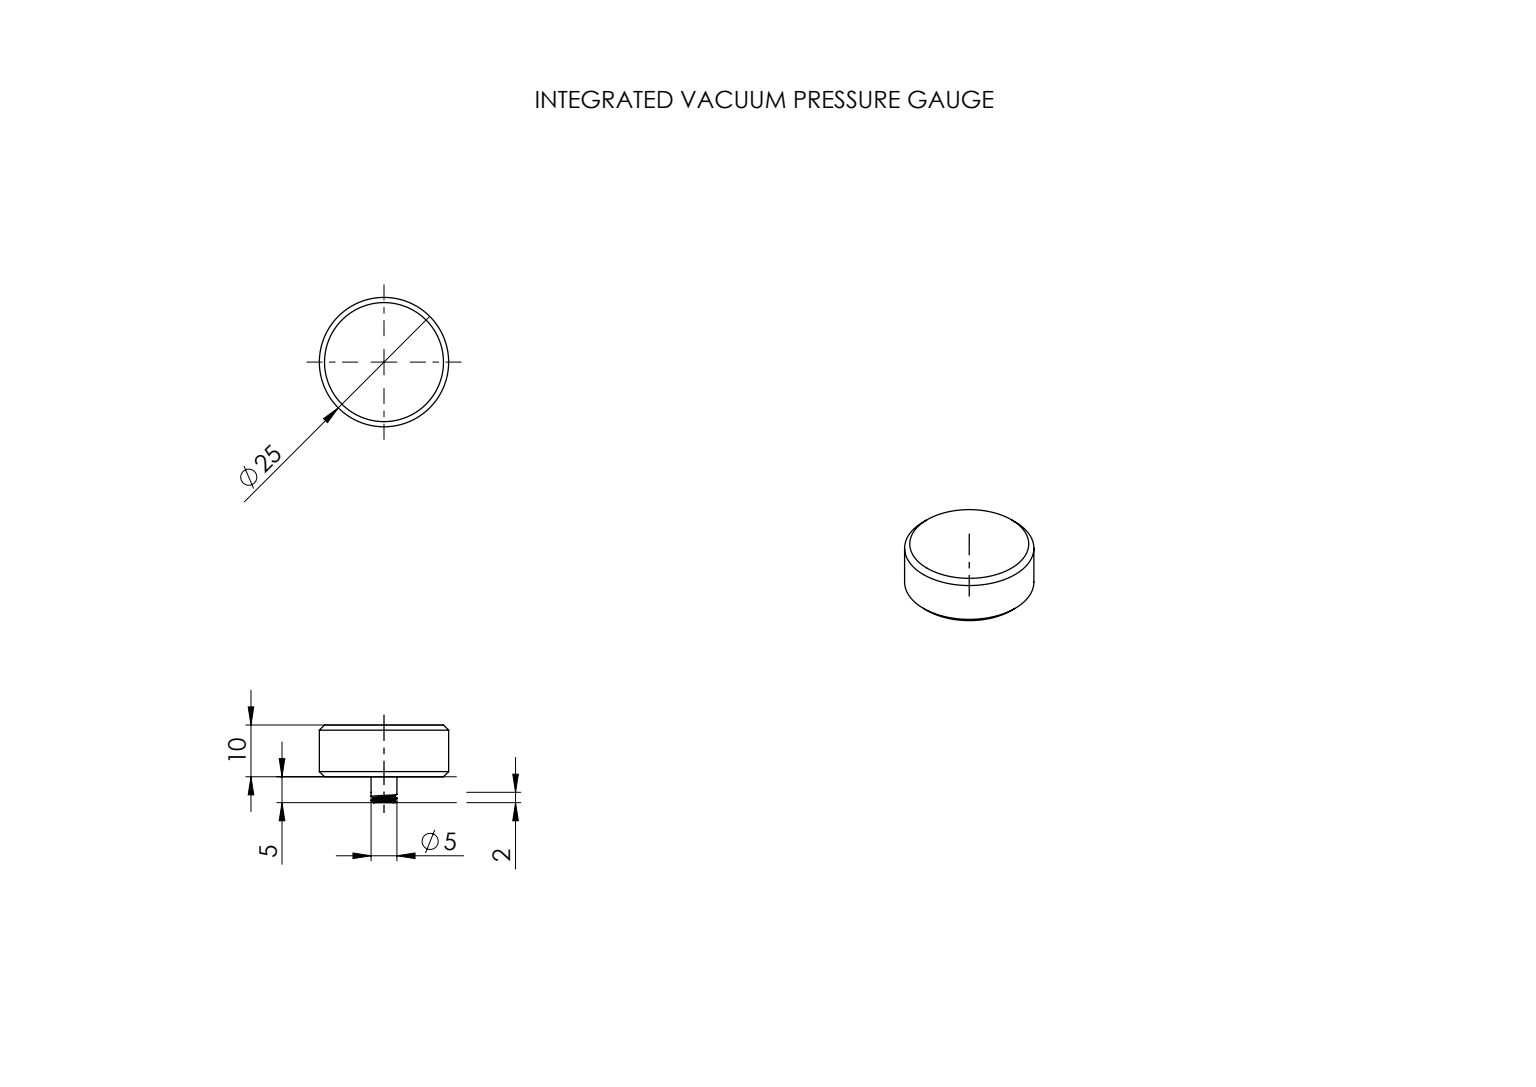
ISO-10303-21;
HEADER;
FILE_DESCRIPTION (('STEP AP214'),
    '1' );
FILE_NAME ('Integrated Vacuum Pressure Gauge.step',
    '2026-10-01T14:18:43',
    ( '' ),
    ( '' ),
    'SwSTEP 2.0',
    'SolidWorks 2026',
    '' );
FILE_SCHEMA (( 'AUTOMOTIVE_DESIGN' ));
ENDSEC;

DATA;
#26=CARTESIAN_POINT ( 'NONE',  ( 99.99999999999998579, 130.0000000000000000, 0.5000000000000034417 ) ) ;
#35=CARTESIAN_POINT ( 'NONE',  ( 102.0669872999999797, 124.3500000010924822, -9.794112055954760458E-15 ) ) ;
#135=CARTESIAN_POINT ( 'NONE',  ( 97.93294022916485631, 122.9999999999999858, -0.1348184704668160261 ) ) ;
#178=CARTESIAN_POINT ( 'NONE',  ( 101.4615807364564546, 124.2500000010924737, 1.461580736456455476 ) ) ;
#224=CYLINDRICAL_SURFACE ( 'NONE', #5646, 2.500000000000008882 ) ;
#256=ADVANCED_FACE ( 'NONE', ( #12743 ), #3942, .F. ) ;
#307=AXIS2_PLACEMENT_3D ( 'NONE', #10055, #1393, #9916 ) ;
#308=CARTESIAN_POINT ( 'NONE',  ( 97.93301270000000613, 124.7500000010924737, -9.540979117872439019E-15 ) ) ;
#319=CARTESIAN_POINT ( 'NONE',  ( 98.53841926354351699, 124.6500000010924651, -1.461580736456474794 ) ) ;
#324=EDGE_CURVE ( 'NONE', #25689, #13199, #21050, .T. ) ;
#329=ORIENTED_EDGE ( 'NONE', *, *, #20493, .F. ) ;
#336=AXIS2_PLACEMENT_3D ( 'NONE', #4217, #10471, #27744 ) ;
#342=EDGE_LOOP ( 'NONE', ( #1311, #13880, #16852, #27004 ) ) ;
#449=CARTESIAN_POINT ( 'NONE',  ( 97.93301269999999192, 124.7000000010924623, -0.8561741729129505041 ) ) ;
#463=CARTESIAN_POINT ( 'NONE',  ( 101.4615807364564546, 124.4500000010924765, -1.461580736456474794 ) ) ;
#487=VERTEX_POINT ( 'NONE', #17746 ) ;
#496=CARTESIAN_POINT ( 'NONE',  ( 97.50000000000000000, 124.9500000000000028, -1.035533905932742416 ) ) ;
#513=PLANE ( 'NONE',  #11990 ) ;
#550=CARTESIAN_POINT ( 'NONE',  ( 97.93301270000000613, 124.5500000010924850, -9.540979117872439019E-15 ) ) ;
#565=ORIENTED_EDGE ( 'NONE', *, *, #12281, .F. ) ;
#566=CARTESIAN_POINT ( 'NONE',  ( 98.35496906260777905, 122.9999999999999858, -1.258827244710729154 ) ) ;
#572=CARTESIAN_POINT ( 'NONE',  ( 101.4674565229751693, 123.0000000000000568, 1.992898914349557682 ) ) ;
#581=AXIS2_PLACEMENT_3D ( 'NONE', #23300, #18317, #25016 ) ;
#603=ORIENTED_EDGE ( 'NONE', *, *, #9339, .T. ) ;
#604=CYLINDRICAL_SURFACE ( 'NONE', #14088, 10.50000000000001599 ) ;
#694=CARTESIAN_POINT ( 'NONE',  ( 99.99999999999998579, 123.9500000010924765, 2.066987299999980099 ) ) ;
#707=CARTESIAN_POINT ( 'NONE',  ( 99.99999999999998579, 123.7000000021849502, 2.499999999999978684 ) ) ;
#748=PRESENTATION_STYLE_ASSIGNMENT (( #20411 ) ) ;
#759=AXIS2_PLACEMENT_3D ( 'NONE', #7749, #5760, #14289 ) ;
#774=AXIS2_PLACEMENT_3D ( 'NONE', #17038, #5950, #27753 ) ;
#782=CARTESIAN_POINT ( 'NONE',  ( 100.8561741729129295, 123.2000000010924765, 2.066987299999979211 ) ) ;
#825=ORIENTED_EDGE ( 'NONE', *, *, #22272, .F. ) ;
#831=PRODUCT_DEFINITION_SHAPE ( 'NONE', 'NONE',  #10642 ) ;
#841=CARTESIAN_POINT ( 'NONE',  ( 98.53841926354351699, 123.6500000010924794, -1.461580736456474794 ) ) ;
#884=DIRECTION ( 'NONE',  ( 0.000000000000000000, 1.000000000000000000, 0.000000000000000000 ) ) ;
#904=ORIENTED_EDGE ( 'NONE', *, *, #5003, .F. ) ;
#925=CARTESIAN_POINT ( 'NONE',  ( 100.8561741729129153, 122.7000000010924623, -2.066987299999999195 ) ) ;
#958=AXIS2_PLACEMENT_3D ( 'NONE', #9694, #13952, #26961 ) ;
#964=EDGE_LOOP ( 'NONE', ( #1933, #20630, #27300, #22886 ) ) ;
#1009=LINE ( 'NONE', #1284, #19265 ) ;
#1014=ORIENTED_EDGE ( 'NONE', *, *, #14713, .T. ) ;
#1024=CARTESIAN_POINT ( 'NONE',  ( 97.50000000000000000, 123.4500000021849502, -1.035533905932742416 ) ) ;
#1028=CARTESIAN_POINT ( 'NONE',  ( 97.93301269999999192, 123.2000000010924765, 0.8561741729129329626 ) ) ;
#1035=DIRECTION ( 'NONE',  ( -0.000000000000000000, -1.000000000000000000, -0.000000000000000000 ) ) ;
#1068=CARTESIAN_POINT ( 'NONE',  ( 102.4999999999999858, 123.1000000021849416, -9.847140817659276890E-15 ) ) ;
#1081=CARTESIAN_POINT ( 'NONE',  ( 99.99999999999998579, 123.9500000010924765, 2.066987299999980099 ) ) ;
#1124=CARTESIAN_POINT ( 'NONE',  ( 102.0669872999999939, 124.2000000010924907, -0.8561741729129507261 ) ) ;
#1164=LINE ( 'NONE', #26817, #17544 ) ;
#1165=CARTESIAN_POINT ( 'NONE',  ( 97.50000000000000000, 123.5000000021849615, -9.540979117872439019E-15 ) ) ;
#1168=CARTESIAN_POINT ( 'NONE',  ( 98.96446609406727646, 123.5499999999999972, 2.499999999999977796 ) ) ;
#1210=CARTESIAN_POINT ( 'NONE',  ( 98.53841926354351699, 124.4500000010924765, -1.461580736456474794 ) ) ;
#1252=DIRECTION ( 'NONE',  ( 0.000000000000000000, 1.000000000000000000, 0.000000000000000000 ) ) ;
#1260=CARTESIAN_POINT ( 'NONE',  ( 97.93301269999999192, 122.9000000010924936, -0.8561741729129505041 ) ) ;
#1284=CARTESIAN_POINT ( 'NONE',  ( 99.99999999999998579, 128.0000000000000000, 0.5000000000000034417 ) ) ;
#1296=( BOUNDED_CURVE ( )  B_SPLINE_CURVE ( 2, ( #5886, #1472, #21125, #8006, #14273 ),
 .UNSPECIFIED., .F., .F. ) 
 B_SPLINE_CURVE_WITH_KNOTS ( ( 3, 2, 3 ),
 ( 0.7499999999999997780, 0.7916666666666665186, 0.8333333333333333703 ),
 .UNSPECIFIED. ) 
 CURVE ( )  GEOMETRIC_REPRESENTATION_ITEM ( )  RATIONAL_B_SPLINE_CURVE ( ( 1.000000000000000444, 0.9238795325112862944, 1.000000000000000000, 0.9238795325112867385, 1.000000000000000000 ) ) 
 REPRESENTATION_ITEM ( '' )  );
#1299=CARTESIAN_POINT ( 'NONE',  ( 98.96446609406727646, 124.3499999999999943, 2.499999999999977796 ) ) ;
#1311=ORIENTED_EDGE ( 'NONE', *, *, #23920, .F. ) ;
#1314=PRODUCT_DEFINITION_FORMATION_WITH_SPECIFIED_SOURCE ( 'ANY', '', #11245, .NOT_KNOWN. ) ;
#1315=CARTESIAN_POINT ( 'NONE',  ( 97.50000000000000000, 124.3000000021849587, -9.540979117872439019E-15 ) ) ;
#1333=FACE_OUTER_BOUND ( 'NONE', #21397, .T. ) ;
#1345=CARTESIAN_POINT ( 'NONE',  ( 97.50000000000000000, 122.7000000021849502, -9.540979117872439019E-15 ) ) ;
#1393=DIRECTION ( 'NONE',  ( 0.000000000000000000, 1.000000000000000000, 0.000000000000000000 ) ) ;
#1394=ADVANCED_FACE ( 'NONE', ( #10481 ), #18907, .T. ) ;
#1400=CARTESIAN_POINT ( 'NONE',  ( 97.93301269999999192, 123.9000000010924794, -0.8561741729129505041 ) ) ;
#1402=CONICAL_SURFACE ( 'NONE', #958, 12.50000000000001599, 0.7853981633974491672 ) ;
#1438=CARTESIAN_POINT ( 'NONE',  ( 99.99999999999998579, 123.3000000021849587, -2.499999999999997780 ) ) ;
#1439=FACE_OUTER_BOUND ( 'NONE', #2427, .T. ) ;
#1441=CARTESIAN_POINT ( 'NONE',  ( 101.7677669529663547, 123.8999999999999915, -1.767766952966370209 ) ) ;
#1472=CARTESIAN_POINT ( 'NONE',  ( 101.0355339059327235, 123.1500000000000057, -2.500000000000001776 ) ) ;
#1539=CARTESIAN_POINT ( 'NONE',  ( 100.8561741729129295, 124.2000000010924907, 2.066987299999979211 ) ) ;
#1546=ORIENTED_EDGE ( 'NONE', *, *, #12281, .T. ) ;
#1562=ORIENTED_EDGE ( 'NONE', *, *, #19274, .F. ) ;
#1577=CARTESIAN_POINT ( 'NONE',  ( 98.23223304703363112, 123.6000000021849416, 1.767766952966351557 ) ) ;
#1582=CARTESIAN_POINT ( 'NONE',  ( 99.99999999999998579, 124.3999999999999915, 2.499999999999978684 ) ) ;
#1590=CARTESIAN_POINT ( 'NONE',  ( 99.99999999999998579, 130.0000000000000000, -5.204170427930421283E-15 ) ) ;
#1596=VERTEX_POINT ( 'NONE', #7017 ) ;
#1625=CARTESIAN_POINT ( 'NONE',  ( 102.0541222904681575, 123.0000000000000142, -1.218761725175215416 ) ) ;
#1628=ORIENTED_EDGE ( 'NONE', *, *, #5003, .T. ) ;
#1713=DIRECTION ( 'NONE',  ( 0.000000000000000000, 0.000000000000000000, -1.000000000000000000 ) ) ;
#1768=DIRECTION ( 'NONE',  ( 1.000000000000000000, 0.000000000000000000, -0.000000000000000000 ) ) ;
#1784=CARTESIAN_POINT ( 'NONE',  ( 99.99999999999998579, 128.0000000000000000, -5.204170427930421283E-15 ) ) ;
#1812=CARTESIAN_POINT ( 'NONE',  ( 102.0669872999999797, 122.7500000010924737, -9.794112055954760458E-15 ) ) ;
#1875=VERTEX_POINT ( 'NONE', #26 ) ;
#1904=CARTESIAN_POINT ( 'NONE',  ( 98.41882588794221931, 123.0000000000000284, 1.462731629774626230 ) ) ;
#1933=ORIENTED_EDGE ( 'NONE', *, *, #21365, .F. ) ;
#2035=CARTESIAN_POINT ( 'NONE',  ( 99.14382582708708469, 123.8000000010924566, -2.066987299999998751 ) ) ;
#2047=CIRCLE ( 'NONE', #21610, 11.50000000000001421 ) ;
#2068=ORIENTED_EDGE ( 'NONE', *, *, #19448, .F. ) ;
#2138=CARTESIAN_POINT ( 'NONE',  ( 102.4999999999999858, 123.7999999999999972, -9.847140817659276890E-15 ) ) ;
#2210=DIRECTION ( 'NONE',  ( -0.000000000000000000, -1.000000000000000000, -0.000000000000000000 ) ) ;
#2260=DIRECTION ( 'NONE',  ( 0.000000000000000000, -1.000000000000000000, 0.000000000000000000 ) ) ;
#2283=CARTESIAN_POINT ( 'NONE',  ( 99.20899822134843760, 123.0000000000000000, -1.909647267044714436 ) ) ;
#2286=ORIENTED_EDGE ( 'NONE', *, *, #22272, .T. ) ;
#2322=CARTESIAN_POINT ( 'NONE',  ( 98.53841926354351699, 124.0500000010924708, 1.461580736456455920 ) ) ;
#2342=ADVANCED_FACE ( 'NONE', ( #12099 ), #5329, .T. ) ;
#2343=ORIENTED_EDGE ( 'NONE', *, *, #5269, .T. ) ;
#2348=CARTESIAN_POINT ( 'NONE',  ( 101.0355339059327235, 124.4499999999999744, 2.499999999999974687 ) ) ;
#2368=CARTESIAN_POINT ( 'NONE',  ( 99.99999999999998579, 123.6000000000000085, 2.499999999999978684 ) ) ;
#2391=DIRECTION ( 'NONE',  ( 0.000000000000000000, 1.000000000000000000, 0.000000000000000000 ) ) ;
#2401=DIRECTION ( 'NONE',  ( -0.000000000000000000, -1.000000000000000000, -0.000000000000000000 ) ) ;
#2427=EDGE_LOOP ( 'NONE', ( #15836, #21135, #8076, #4426 ) ) ;
#2436=DIRECTION ( 'NONE',  ( 0.000000000000000000, 1.000000000000000000, 0.000000000000000000 ) ) ;
#2550=DIRECTION ( 'NONE',  ( -0.8660254037844380415, 0.5000000000000013323, 0.000000000000000000 ) ) ;
#2577=( BOUNDED_CURVE ( )  B_SPLINE_CURVE ( 2, ( #13774, #22212, #20358, #26925, #7084, #3255, #11781 ),
 .UNSPECIFIED., .F., .T. ) 
 B_SPLINE_CURVE_WITH_KNOTS ( ( 3, 2, 2, 3 ),
 ( 0.4166666666666666297, 0.4583333333333332593, 0.5000000000000000000, 0.5416666676520737189 ),
 .UNSPECIFIED. ) 
 CURVE ( )  GEOMETRIC_REPRESENTATION_ITEM ( )  RATIONAL_B_SPLINE_CURVE ( ( 1.000000000000000000, 0.9238795325112866275, 1.000000000000000000, 0.9238795325112867385, 1.000000000000000000, 0.9238795325112867385, 1.000000000000000000 ) ) 
 REPRESENTATION_ITEM ( '' )  );
#2616=( BOUNDED_CURVE ( )  B_SPLINE_CURVE ( 2, ( #27650, #12227, #1577, #16390, #1165, #1024, #16532, #27101, #1438 ),
 .UNSPECIFIED., .F., .T. ) 
 B_SPLINE_CURVE_WITH_KNOTS ( ( 3, 2, 2, 2, 3 ),
 ( 0.2500000000000004441, 0.2916666666666670182, 0.3333333333333334814, 0.3750000000000000555, 0.4166666666666666297 ),
 .UNSPECIFIED. ) 
 CURVE ( )  GEOMETRIC_REPRESENTATION_ITEM ( )  RATIONAL_B_SPLINE_CURVE ( ( 0.9999999999999992228, 0.9238795325112875156, 1.000000000000000000, 0.9238795325112867385, 1.000000000000000000, 0.9238795325112867385, 1.000000000000000000, 0.9238795325112868495, 0.9999999999999998890 ) ) 
 REPRESENTATION_ITEM ( '' )  );
#2621=VERTEX_POINT ( 'NONE', #25441 ) ;
#2644=CARTESIAN_POINT ( 'NONE',  ( 97.93301270000000613, 123.7000000010924765, -0.8561741729129506151 ) ) ;
#2646=CARTESIAN_POINT ( 'NONE',  ( 99.99999999999998579, 123.7000000021849502, 2.499999999999978684 ) ) ;
#2688=CARTESIAN_POINT ( 'NONE',  ( 99.99999999999998579, 124.3500000010924822, -2.066987299999998751 ) ) ;
#2696=ADVANCED_FACE ( 'NONE', ( #12164, #25295 ), #20892, .F. ) ;
#2704=CARTESIAN_POINT ( 'NONE',  ( 99.99999999999998579, 137.0000000000000000, -12.50000000000002132 ) ) ;
#2711=CARTESIAN_POINT ( 'NONE',  ( 100.4037632238151048, 123.0000000000000426, 2.336451931449787356 ) ) ;
#2726=ADVANCED_FACE ( 'NONE', ( #2770 ), #22578, .T. ) ;
#2743=SURFACE_STYLE_FILL_AREA ( #7568 ) ;
#2770=FACE_OUTER_BOUND ( 'NONE', #10578, .T. ) ;
#2785=CARTESIAN_POINT ( 'NONE',  ( 97.93301270000000613, 123.7500000010924879, -9.540979117872439019E-15 ) ) ;
#2789=CARTESIAN_POINT ( 'NONE',  ( 99.99999999999998579, 128.0000000000000000, -5.204170427930421283E-15 ) ) ;
#2906=CARTESIAN_POINT ( 'NONE',  ( 99.14382582708707048, 123.6000000010924680, -2.066987299999999195 ) ) ;
#2920=CARTESIAN_POINT ( 'NONE',  ( 101.0355339059327093, 124.0500000021849445, -2.500000000000002665 ) ) ;
#2958=CARTESIAN_POINT ( 'NONE',  ( 100.8561741729129295, 124.0000000010925021, 2.066987299999979211 ) ) ;
#3051=CARTESIAN_POINT ( 'NONE',  ( 97.93301269999999192, 123.0000000010925163, 0.8561741729129329626 ) ) ;
#3066=CARTESIAN_POINT ( 'NONE',  ( 99.99999999999998579, 123.5500000010924850, -2.066987299999998751 ) ) ;
#3068=CARTESIAN_POINT ( 'NONE',  ( 101.7677669529663547, 123.8000000021849587, 1.767766952966350891 ) ) ;
#3075=EDGE_CURVE ( 'NONE', #6277, #13578, #23004, .T. ) ;
#3109=CARTESIAN_POINT ( 'NONE',  ( 99.99999999999998579, 123.1500000010924794, 2.066987299999980099 ) ) ;
#3119=EDGE_CURVE ( 'NONE', #23148, #6493, #15165, .T. ) ;
#3137=CIRCLE ( 'NONE', #13520, 0.5000000000000086597 ) ;
#3142=VERTEX_POINT ( 'NONE', #19836 ) ;
#3153=CARTESIAN_POINT ( 'NONE',  ( 102.0669872999999797, 122.7500000010924737, -9.794112055954760458E-15 ) ) ;
#3163=ORIENTED_EDGE ( 'NONE', *, *, #26053, .F. ) ;
#3170=EDGE_CURVE ( 'NONE', #4566, #13199, #10297, .T. ) ;
#3191=CARTESIAN_POINT ( 'NONE',  ( 102.4999999999999716, 122.3500000021849701, -1.035533905932742638 ) ) ;
#3210=DIRECTION ( 'NONE',  ( 0.000000000000000000, 0.000000000000000000, 1.000000000000000000 ) ) ;
#3215=( NAMED_UNIT ( * ) SI_UNIT ( $, .STERADIAN. ) SOLID_ANGLE_UNIT ( ) );
#3250=CARTESIAN_POINT ( 'NONE',  ( 99.99999999999998579, 138.0000000000000000, -5.204170427930421283E-15 ) ) ;
#3255=CARTESIAN_POINT ( 'NONE',  ( 102.4999999999999858, 123.0500000021849587, 1.035533905932722876 ) ) ;
#3271=ORIENTED_EDGE ( 'NONE', *, *, #20663, .F. ) ;
#3293=CARTESIAN_POINT ( 'NONE',  ( 97.50000000000000000, 124.2000000000000028, -9.540979117872439019E-15 ) ) ;
#3332=CARTESIAN_POINT ( 'NONE',  ( 102.0669872999999939, 123.3000000010924850, 0.8561741729129311862 ) ) ;
#3342=CIRCLE ( 'NONE', #13770, 12.50000000000001599 ) ;
#3344=ORIENTED_EDGE ( 'NONE', *, *, #18362, .T. ) ;
#3345=DIRECTION ( 'NONE',  ( 0.000000000000000000, 0.000000000000000000, 1.000000000000000000 ) ) ;
#3354=CYLINDRICAL_SURFACE ( 'NONE', #28022, 0.5000000000000086597 ) ;
#3381=CARTESIAN_POINT ( 'NONE',  ( 99.99999999999998579, 124.5500000010924708, -2.066987299999998751 ) ) ;
#3427=CARTESIAN_POINT ( 'NONE',  ( 97.50000000000000000, 124.2500000000000000, 1.035533905932725096 ) ) ;
#3437=DIRECTION ( 'NONE',  ( 0.000000000000000000, -0.000000000000000000, 1.000000000000000000 ) ) ;
#3444=B_SPLINE_CURVE_WITH_KNOTS ( 'NONE', 3,
 ( #16511, #21484, #14629, #8089, #25204, #3821 ),
 .UNSPECIFIED., .F., .F.,
 ( 4, 2, 4 ),
 ( 0.1250000000000000000, 0.1875000000000000000, 0.2500000000000000000 ),
 .UNSPECIFIED. ) ;
#3461=DIRECTION ( 'NONE',  ( 0.000000000000000000, 0.000000000000000000, 1.000000000000000000 ) ) ;
#3471=CARTESIAN_POINT ( 'NONE',  ( 102.4999999999999716, 123.0500000021849445, 1.035533905932722876 ) ) ;
#3474=CARTESIAN_POINT ( 'NONE',  ( 99.99999999999998579, 128.0000000000000000, -2.500000000000013767 ) ) ;
#3509=ORIENTED_EDGE ( 'NONE', *, *, #6847, .T. ) ;
#3523=CARTESIAN_POINT ( 'NONE',  ( 101.0355339059327378, 124.0500000021849445, -2.499999999999997780 ) ) ;
#3532=CARTESIAN_POINT ( 'NONE',  ( 100.8561741729129153, 122.7000000010924623, -2.066987299999999195 ) ) ;
#3574=CARTESIAN_POINT ( 'NONE',  ( 97.50000000000000000, 123.3999999999999915, -9.540979117872439019E-15 ) ) ;
#3578=DIRECTION ( 'NONE',  ( 0.000000000000000000, 0.000000000000000000, -1.000000000000000000 ) ) ;
#3582=FACE_OUTER_BOUND ( 'NONE', #18019, .T. ) ;
#3624=ORIENTED_EDGE ( 'NONE', *, *, #10051, .F. ) ;
#3626=PLANE ( 'NONE',  #23713 ) ;
#3639=SURFACE_STYLE_FILL_AREA ( #23163 ) ;
#3662=CARTESIAN_POINT ( 'NONE',  ( 99.99999999999998579, 123.0000000000000000, -5.204170427930421283E-15 ) ) ;
#3665=CARTESIAN_POINT ( 'NONE',  ( 98.23223304703363112, 123.6000000021849416, 1.767766952966351557 ) ) ;
#3674=CARTESIAN_POINT ( 'NONE',  ( 97.93301270000000613, 122.9500000010924765, -9.540979117872439019E-15 ) ) ;
#3713=CARTESIAN_POINT ( 'NONE',  ( 99.99999999999998579, 122.9500000010924765, -2.066987299999998751 ) ) ;
#3728=ORIENTED_EDGE ( 'NONE', *, *, #3075, .T. ) ;
#3804=CARTESIAN_POINT ( 'NONE',  ( 99.14382582708707048, 123.3000000010924708, 2.066987299999979211 ) ) ;
#3821=CARTESIAN_POINT ( 'NONE',  ( 102.4999999999999858, 123.0000000000000000, -8.724596124144689908E-15 ) ) ;
#3824=VERTEX_POINT ( 'NONE', #4002 ) ;
#3840=EDGE_CURVE ( 'NONE', #16572, #23831, #15188, .T. ) ;
#3879=CARTESIAN_POINT ( 'NONE',  ( 97.50000000000000000, 124.6500000010924651, -9.540979117872439019E-15 ) ) ;
#3893=CARTESIAN_POINT ( 'NONE',  ( 100.4820290753432488, 123.0000000000000284, -2.155989633091683011 ) ) ;
#3936=PLANE ( 'NONE',  #11130 ) ;
#3942=CYLINDRICAL_SURFACE ( 'NONE', #336, 10.50000000000001599 ) ;
#3956=ADVANCED_FACE ( 'NONE', ( #22873 ), #25655, .F. ) ;
#4002=CARTESIAN_POINT ( 'NONE',  ( 99.99999999999998579, 136.0000000000000000, 10.50000000000001066 ) ) ;
#4026=CARTESIAN_POINT ( 'NONE',  ( 102.4999999999999858, 123.7500000000000142, 1.035533905932722876 ) ) ;
#4104=ORIENTED_EDGE ( 'NONE', *, *, #12527, .F. ) ;
#4175=CARTESIAN_POINT ( 'NONE',  ( 100.1069863019943114, 123.0000000000000000, -2.169275729499147598 ) ) ;
#4196=CARTESIAN_POINT ( 'NONE',  ( 99.99999999999998579, 124.3999999999999915, 2.499999999999978684 ) ) ;
#4217=CARTESIAN_POINT ( 'NONE',  ( 99.99999999999998579, 138.0000000000000000, -5.204170427930421283E-15 ) ) ;
#4260=CARTESIAN_POINT ( 'NONE',  ( 101.0355339059327378, 123.1499999999999915, -2.499999999999997780 ) ) ;
#4261=ADVANCED_FACE ( 'NONE', ( #6651 ), #28189, .T. ) ;
#4270=CARTESIAN_POINT ( 'NONE',  ( 102.4999999999999858, 123.8500000000000085, -1.035533905932742638 ) ) ;
#4278=ORIENTED_EDGE ( 'NONE', *, *, #26223, .T. ) ;
#4279=EDGE_CURVE ( 'NONE', #13199, #4566, #7028, .T. ) ;
#4335=CARTESIAN_POINT ( 'NONE',  ( 102.4999999999999858, 124.6500000000000057, -1.035533905932742638 ) ) ;
#4383=CARTESIAN_POINT ( 'NONE',  ( 99.99999999999998579, 128.0000000000000000, -2.500000000000013767 ) ) ;
#4391=CIRCLE ( 'NONE', #759, 11.50000000000001776 ) ;
#4414=CARTESIAN_POINT ( 'NONE',  ( 98.14149105024047515, 122.9999999999999432, -0.9146729478038871930 ) ) ;
#4426=ORIENTED_EDGE ( 'NONE', *, *, #20131, .F. ) ;
#4455=DIRECTION ( 'NONE',  ( 0.000000000000000000, 0.000000000000000000, 1.000000000000000000 ) ) ;
#4527=DIRECTION ( 'NONE',  ( 0.000000000000000000, 0.000000000000000000, 1.000000000000000000 ) ) ;
#4548=ADVANCED_FACE ( 'NONE', ( #10322, #23046 ), #14327, .F. ) ;
#4552=CARTESIAN_POINT ( 'NONE',  ( 101.7677669529663547, 123.7000000000000028, 1.767766952966350891 ) ) ;
#4566=VERTEX_POINT ( 'NONE', #27466 ) ;
#4591=CARTESIAN_POINT ( 'NONE',  ( 98.53841926354351699, 123.2500000010924737, 1.461580736456455920 ) ) ;
#4605=ADVANCED_FACE ( 'NONE', ( #12180 ), #3936, .F. ) ;
#4646=CARTESIAN_POINT ( 'NONE',  ( 97.50000000000000000, 124.2000000000000028, -9.540979117872439019E-15 ) ) ;
#4724=CARTESIAN_POINT ( 'NONE',  ( 99.14382582708707048, 124.6000000010924822, -2.066987299999999195 ) ) ;
#4736=CARTESIAN_POINT ( 'NONE',  ( 97.93301270000000613, 124.7000000010924765, -0.8561741729129506151 ) ) ;
#4779=CARTESIAN_POINT ( 'NONE',  ( 98.24769277278620905, 123.0259891538152743, 1.170854245699148866 ) ) ;
#4781=CARTESIAN_POINT ( 'NONE',  ( 102.4999999999999858, 123.9500000021849502, -1.035533905932742638 ) ) ;
#4786=DIRECTION ( 'NONE',  ( 0.000000000000000000, 1.000000000000000000, 0.000000000000000000 ) ) ;
#4806=CARTESIAN_POINT ( 'NONE',  ( 99.99999999999998579, 136.0000000000000000, -5.204170427930421283E-15 ) ) ;
#4848=CARTESIAN_POINT ( 'NONE',  ( 98.54104284345754650, 123.0000000000000426, 1.608754092638752242 ) ) ;
#4871=DIRECTION ( 'NONE',  ( 0.000000000000000000, 0.000000000000000000, 1.000000000000000000 ) ) ;
#4882=CARTESIAN_POINT ( 'NONE',  ( 97.93301270000000613, 124.0000000010924879, 0.8561741729129328515 ) ) ;
#4890=EDGE_LOOP ( 'NONE', ( #19676, #17943 ) ) ;
#4925=CARTESIAN_POINT ( 'NONE',  ( 102.0669873000000081, 123.3000000010924850, 0.8561741729129311862 ) ) ;
#4967=CIRCLE ( 'NONE', #12217, 10.50000000000001599 ) ;
#4971=FACE_OUTER_BOUND ( 'NONE', #16611, .T. ) ;
#5003=EDGE_CURVE ( 'NONE', #6030, #10914, #12276, .T. ) ;
#5049=DIRECTION ( 'NONE',  ( 0.000000000000000000, 0.000000000000000000, -1.000000000000000000 ) ) ;
#5052=CARTESIAN_POINT ( 'NONE',  ( 99.99999999999998579, 123.5500000010924850, -2.066987299999998751 ) ) ;
#5065=CARTESIAN_POINT ( 'NONE',  ( 97.93301270000000613, 124.5500000010924850, -9.540979117872439019E-15 ) ) ;
#5089=DIRECTION ( 'NONE',  ( 0.000000000000000000, 0.000000000000000000, 1.000000000000000000 ) ) ;
#5193=CARTESIAN_POINT ( 'NONE',  ( 99.14382582708707048, 123.9000000010924794, 2.066987299999979211 ) ) ;
#5203=ORIENTED_EDGE ( 'NONE', *, *, #26645, .T. ) ;
#5249=CARTESIAN_POINT ( 'NONE',  ( 97.93301269999999192, 123.7000000010924765, -0.8561741729129505041 ) ) ;
#5267=ORIENTED_EDGE ( 'NONE', *, *, #12792, .T. ) ;
#5269=EDGE_CURVE ( 'NONE', #18860, #22175, #2047, .T. ) ;
#5292=CARTESIAN_POINT ( 'NONE',  ( 97.50000000000000000, 125.0000000000000000, -9.540979117872439019E-15 ) ) ;
#5329=CONICAL_SURFACE ( 'NONE', #11688, 11.50000000000001776, 0.7853981633974473908 ) ;
#5335=CARTESIAN_POINT ( 'NONE',  ( 102.0669872999999939, 124.2000000010924907, -0.8561741729129507261 ) ) ;
#5349=CARTESIAN_POINT ( 'NONE',  ( 98.53841926354351699, 123.8500000010924680, 1.461580736456455920 ) ) ;
#5375=ORIENTED_EDGE ( 'NONE', *, *, #22515, .T. ) ;
#5393=CARTESIAN_POINT ( 'NONE',  ( 98.53841926354351699, 123.0500000010924850, 1.461580736456455920 ) ) ;
#5436=CARTESIAN_POINT ( 'NONE',  ( 102.0669872999999939, 123.6000000010924680, -0.8561741729129507261 ) ) ;
#5447=ORIENTED_EDGE ( 'NONE', *, *, #15750, .F. ) ;
#5475=CARTESIAN_POINT ( 'NONE',  ( 98.53841926354351699, 123.8500000010924680, 1.461580736456455920 ) ) ;
#5482=ORIENTED_EDGE ( 'NONE', *, *, #20131, .T. ) ;
#5499=VECTOR ( 'NONE', #8282, 1000.000000000000000 ) ;
#5503=FACE_OUTER_BOUND ( 'NONE', #18514, .T. ) ;
#5505=EDGE_CURVE ( 'NONE', #8833, #9543, #18765, .T. ) ;
#5509=ADVANCED_FACE ( 'NONE', ( #23049 ), #15019, .T. ) ;
#5579=CARTESIAN_POINT ( 'NONE',  ( 100.8561741729129153, 123.7000000010924765, -2.066987299999999195 ) ) ;
#5591=FILL_AREA_STYLE_COLOUR ( '', #9978 ) ;
#5617=CARTESIAN_POINT ( 'NONE',  ( 100.8561741729129153, 124.3000000010924708, -2.066987299999999195 ) ) ;
#5646=AXIS2_PLACEMENT_3D ( 'NONE', #2789, #9471, #11168 ) ;
#5665=CARTESIAN_POINT ( 'NONE',  ( 97.50000000000000000, 123.5000000021849615, -9.540979117872439019E-15 ) ) ;
#5673=CARTESIAN_POINT ( 'NONE',  ( 102.0669872999999939, 124.4000000010924651, -0.8561741729129507261 ) ) ;
#5716=CARTESIAN_POINT ( 'NONE',  ( 99.14382582708707048, 123.0000000010925021, -2.066987299999999195 ) ) ;
#5721=DIRECTION ( 'NONE',  ( 0.000000000000000000, -1.000000000000000000, 0.000000000000000000 ) ) ;
#5760=DIRECTION ( 'NONE',  ( 0.000000000000000000, 1.000000000000000000, 0.000000000000000000 ) ) ;
#5765=FACE_OUTER_BOUND ( 'NONE', #20936, .T. ) ;
#5810=CARTESIAN_POINT ( 'NONE',  ( 101.4615807364564546, 123.6500000010924651, -1.461580736456474794 ) ) ;
#5850=CARTESIAN_POINT ( 'NONE',  ( 99.99999999999998579, 123.3500000010924680, 2.066987299999980099 ) ) ;
#5853=SHAPE_DEFINITION_REPRESENTATION ( #831, #10045 ) ;
#5886=CARTESIAN_POINT ( 'NONE',  ( 99.99999999999998579, 123.2000000000000028, -2.499999999999997780 ) ) ;
#5901=CARTESIAN_POINT ( 'NONE',  ( 102.2498298612819525, 123.0000000000000284, -0.9005770716734564640 ) ) ;
#5950=DIRECTION ( 'NONE',  ( -0.000000000000000000, -1.000000000000000000, -0.000000000000000000 ) ) ;
#6030=VERTEX_POINT ( 'NONE', #19225 ) ;
#6035=CARTESIAN_POINT ( 'NONE',  ( 101.5243464873929042, 123.0000000000000000, -1.749128039131298884 ) ) ;
#6038=ORIENTED_EDGE ( 'NONE', *, *, #21365, .T. ) ;
#6060=DIRECTION ( 'NONE',  ( 0.000000000000000000, -0.000000000000000000, 1.000000000000000000 ) ) ;
#6081=CARTESIAN_POINT ( 'NONE',  ( 101.4615807364564546, 123.4500000010924765, 1.461580736456455476 ) ) ;
#6217=CIRCLE ( 'NONE', #307, 2.500000000000008882 ) ;
#6220=CARTESIAN_POINT ( 'NONE',  ( 101.4615807364564546, 124.2500000010924737, 1.461580736456455476 ) ) ;
#6277=VERTEX_POINT ( 'NONE', #26927 ) ;
#6289=VECTOR ( 'NONE', #13039, 1000.000000000000000 ) ;
#6299=EDGE_LOOP ( 'NONE', ( #5203, #14768, #7767, #13424 ) ) ;
#6303=CARTESIAN_POINT ( 'NONE',  ( 101.1344650075701566, 123.0000000000000426, 2.161518037331323416 ) ) ;
#6325=CARTESIAN_POINT ( 'NONE',  ( 102.4999999999999858, 124.6000000000000085, -9.847140817659276890E-15 ) ) ;
#6354=ORIENTED_EDGE ( 'NONE', *, *, #24509, .T. ) ;
#6442=CARTESIAN_POINT ( 'NONE',  ( 102.0669873000000081, 124.3000000010924708, 0.8561741729129311862 ) ) ;
#6443=CARTESIAN_POINT ( 'NONE',  ( 98.09035273295538104, 123.0000000000000142, 0.7910017786517971050 ) ) ;
#6493=VERTEX_POINT ( 'NONE', #21197 ) ;
#6498=CARTESIAN_POINT ( 'NONE',  ( 99.99999999999998579, 124.3999999999999915, 2.499999999999978684 ) ) ;
#6551=ORIENTED_EDGE ( 'NONE', *, *, #7742, .T. ) ;
#6576=CARTESIAN_POINT ( 'NONE',  ( 99.55174954624675365, 123.0000000000000426, -2.068055351820230481 ) ) ;
#6627=CARTESIAN_POINT ( 'NONE',  ( 98.23223304703363112, 124.1000000000000085, -1.767766952966370209 ) ) ;
#6651=FACE_OUTER_BOUND ( 'NONE', #342, .T. ) ;
#6685=ORIENTED_EDGE ( 'NONE', *, *, #26223, .F. ) ;
#6729=ADVANCED_FACE ( 'NONE', ( #5503 ), #3354, .F. ) ;
#6801=AXIS2_PLACEMENT_3D ( 'NONE', #3250, #27206, #22492 ) ;
#6847=EDGE_CURVE ( 'NONE', #15313, #8172, #15721, .T. ) ;
#6856=CARTESIAN_POINT ( 'NONE',  ( 99.99999999999998579, 124.5500000010924708, -2.066987299999998751 ) ) ;
#6870=AXIS2_PLACEMENT_3D ( 'NONE', #14683, #16706, #3461 ) ;
#6903=CARTESIAN_POINT ( 'NONE',  ( 102.0669873000000081, 124.1000000010924822, 0.8561741729129311862 ) ) ;
#6936=CARTESIAN_POINT ( 'NONE',  ( 99.99999999999998579, 128.0000000000000000, -5.204170427930421283E-15 ) ) ;
#6960=CARTESIAN_POINT ( 'NONE',  ( 101.0355339059327093, 123.6500000000000057, 2.499999999999984457 ) ) ;
#6965=CARTESIAN_POINT ( 'NONE',  ( 98.21999331106005116, 123.0000000000000426, 1.143679003824301876 ) ) ;
#6998=CARTESIAN_POINT ( 'NONE',  ( 99.99999999999998579, 123.3500000010924680, 2.066987299999980099 ) ) ;
#7017=CARTESIAN_POINT ( 'NONE',  ( 99.99999999999998579, 130.0000000000000000, -10.50000000000002132 ) ) ;
#7028=CIRCLE ( 'NONE', #16152, 12.50000000000001599 ) ;
#7073=AXIS2_PLACEMENT_3D ( 'NONE', #18872, #23720, #12576 ) ;
#7084=CARTESIAN_POINT ( 'NONE',  ( 102.4999999999999858, 123.1000000021849416, -9.847140817659276890E-15 ) ) ;
#7103=CARTESIAN_POINT ( 'NONE',  ( 98.14342173294696181, 123.0000000000000426, 0.9730510570952660698 ) ) ;
#7176=CARTESIAN_POINT ( 'NONE',  ( 98.09035273295538104, 123.0000000000000142, 0.7910017786517971050 ) ) ;
#7245=( GEOMETRIC_REPRESENTATION_CONTEXT ( 3 ) GLOBAL_UNCERTAINTY_ASSIGNED_CONTEXT ( ( #12316 ) ) GLOBAL_UNIT_ASSIGNED_CONTEXT ( ( #10162, #18871, #22748 ) ) REPRESENTATION_CONTEXT ( 'NONE', 'WORKASPACE' ) );
#7281=FACE_OUTER_BOUND ( 'NONE', #27266, .T. ) ;
#7312=CARTESIAN_POINT ( 'NONE',  ( 97.93301269999999192, 124.5000000010924879, -0.8561741729129505041 ) ) ;
#7324=CARTESIAN_POINT ( 'NONE',  ( 99.99999999999998579, 123.1500000010924794, 2.066987299999980099 ) ) ;
#7365=CARTESIAN_POINT ( 'NONE',  ( 98.53841926354351699, 124.4500000010924765, -1.461580736456474794 ) ) ;
#7409=CARTESIAN_POINT ( 'NONE',  ( 102.4999999999999716, 124.5500000000000114, 1.035533905932722876 ) ) ;
#7437=AXIS2_PLACEMENT_3D ( 'NONE', #23744, #8768, #17457 ) ;
#7453=CARTESIAN_POINT ( 'NONE',  ( 102.0669872999999797, 122.5500000010924850, -9.794112055954760458E-15 ) ) ;
#7476=SURFACE_STYLE_USAGE ( .BOTH. , #23305 ) ;
#7509=CARTESIAN_POINT ( 'NONE',  ( 99.99999999999998579, 129.0000000000000000, -12.50000000000002132 ) ) ;
#7512=CARTESIAN_POINT ( 'NONE',  ( 101.4615807364564546, 123.4500000010924765, -1.461580736456474794 ) ) ;
#7552=FACE_OUTER_BOUND ( 'NONE', #23998, .T. ) ;
#7556=CARTESIAN_POINT ( 'NONE',  ( 102.0669872999999797, 123.5500000010924708, -9.794112055954760458E-15 ) ) ;
#7568=FILL_AREA_STYLE ('',( #5591 ) ) ;
#7592=EDGE_LOOP ( 'NONE', ( #1014, #4278, #13635, #18831 ) ) ;
#7604=CARTESIAN_POINT ( 'NONE',  ( 101.7677669529663547, 123.2000000021849502, -1.767766952966370209 ) ) ;
#7621=VECTOR ( 'NONE', #28021, 999.9999999999998863 ) ;
#7636=LINE ( 'NONE', #9209, #26683 ) ;
#7659=CIRCLE ( 'NONE', #27256, 0.5000000000000086597 ) ;
#7701=CARTESIAN_POINT ( 'NONE',  ( 99.99999999999998579, 124.7999999999999972, -2.499999999999997780 ) ) ;
#7742=EDGE_CURVE ( 'NONE', #24651, #6493, #23623, .T. ) ;
#7744=CARTESIAN_POINT ( 'NONE',  ( 99.99999999999998579, 123.3000000021849587, -2.499999999999997780 ) ) ;
#7749=CARTESIAN_POINT ( 'NONE',  ( 99.99999999999998579, 138.0000000000000000, -5.204170427930421283E-15 ) ) ;
#7767=ORIENTED_EDGE ( 'NONE', *, *, #27520, .T. ) ;
#7794=CARTESIAN_POINT ( 'NONE',  ( 101.7677669529663547, 123.8000000021849587, 1.767766952966350891 ) ) ;
#7801=CARTESIAN_POINT ( 'NONE',  ( 100.8561741729129153, 123.7000000010924765, -2.066987299999999195 ) ) ;
#7812=CARTESIAN_POINT ( 'NONE',  ( 99.99999999999998579, 128.0000000000000000, -2.500000000000013767 ) ) ;
#7834=DIRECTION ( 'NONE',  ( 0.000000000000000000, 0.000000000000000000, 1.000000000000000000 ) ) ;
#7835=MANIFOLD_SOLID_BREP ( 'Cavity1', #18093 ) ;
#7841=CARTESIAN_POINT ( 'NONE',  ( 98.53841926354351699, 123.2500000010924737, 1.461580736456455920 ) ) ;
#7881=CARTESIAN_POINT ( 'NONE',  ( 97.93301270000000613, 123.7500000010924879, -9.540979117872439019E-15 ) ) ;
#7895=DIRECTION ( 'NONE',  ( 0.000000000000000000, 0.000000000000000000, 1.000000000000000000 ) ) ;
#7926=CARTESIAN_POINT ( 'NONE',  ( 98.23223304703363112, 124.2000000021849502, -1.767766952966370209 ) ) ;
#7934=CARTESIAN_POINT ( 'NONE',  ( 97.93301269999999192, 123.1000000010924822, -0.8561741729129505041 ) ) ;
#7974=CARTESIAN_POINT ( 'NONE',  ( 97.50000000000000000, 123.3499999999999943, -1.035533905932742416 ) ) ;
#8006=CARTESIAN_POINT ( 'NONE',  ( 102.4999999999999858, 123.0500000000000114, -1.035533905932742638 ) ) ;
#8017=ADVANCED_FACE ( 'NONE', ( #7281 ), #604, .F. ) ;
#8023=CARTESIAN_POINT ( 'NONE',  ( 102.4468180503172476, 122.9999999999999574, -0.3717709916353664212 ) ) ;
#8060=DIRECTION ( 'NONE',  ( 0.000000000000000000, 1.000000000000000000, 0.000000000000000000 ) ) ;
#8063=DIRECTION ( 'NONE',  ( -0.000000000000000000, -1.000000000000000000, -0.000000000000000000 ) ) ;
#8070=CARTESIAN_POINT ( 'NONE',  ( 97.93301270000000613, 124.7500000010924737, -9.540979117872439019E-15 ) ) ;
#8072=EDGE_CURVE ( 'NONE', #3824, #18580, #14115, .T. ) ;
#8076=ORIENTED_EDGE ( 'NONE', *, *, #26053, .T. ) ;
#8089=CARTESIAN_POINT ( 'NONE',  ( 102.4349316916707551, 122.9999999999999289, 0.6543697108981973987 ) ) ;
#8165=CARTESIAN_POINT ( 'NONE',  ( 101.2031690377821462, 123.0000000000000000, -1.942071768828401490 ) ) ;
#8172=VERTEX_POINT ( 'NONE', #23489 ) ;
#8210=CARTESIAN_POINT ( 'NONE',  ( 100.8561741729129153, 124.5000000010924737, -2.066987299999999195 ) ) ;
#8219=LINE ( 'NONE', #23207, #14916 ) ;
#8268=ORIENTED_EDGE ( 'NONE', *, *, #25843, .T. ) ;
#8282=DIRECTION ( 'NONE',  ( 0.000000000000000000, -1.000000000000000000, 0.000000000000000000 ) ) ;
#8297=CARTESIAN_POINT ( 'NONE',  ( 98.97035852359087471, 122.9999999999999858, 1.976093766406173735 ) ) ;
#8309=CIRCLE ( 'NONE', #581, 0.5000000000000086597 ) ;
#8348=CARTESIAN_POINT ( 'NONE',  ( 99.99999999999998579, 129.0000000000000000, 12.50000000000001066 ) ) ;
#8353=ORIENTED_EDGE ( 'NONE', *, *, #15195, .T. ) ;
#8481=EDGE_CURVE ( 'NONE', #23831, #15488, #21631, .T. ) ;
#8494=EDGE_LOOP ( 'NONE', ( #5267, #6038 ) ) ;
#8578=CARTESIAN_POINT ( 'NONE',  ( 99.14382582708708469, 124.1000000010924822, 2.066987299999979655 ) ) ;
#8634=CARTESIAN_POINT ( 'NONE',  ( 97.50000000000000000, 124.1499999999999915, -1.035533905932742416 ) ) ;
#8635=CARTESIAN_POINT ( 'NONE',  ( 0.000000000000000000, 0.000000000000000000, 0.000000000000000000 ) ) ;
#8720=CARTESIAN_POINT ( 'NONE',  ( 99.20899822134843760, 123.0000000000000000, -1.909647267044714436 ) ) ;
#8768=DIRECTION ( 'NONE',  ( -0.000000000000000000, -1.000000000000000000, -0.000000000000000000 ) ) ;
#8821=CARTESIAN_POINT ( 'NONE',  ( 97.93315853025627860, 123.0000000000000000, 0.2729566057089571340 ) ) ;
#8833=VERTEX_POINT ( 'NONE', #11899 ) ;
#8860=CARTESIAN_POINT ( 'NONE',  ( 101.4615807364564546, 123.6500000010924651, -1.461580736456474794 ) ) ;
#8878=ORIENTED_EDGE ( 'NONE', *, *, #20853, .F. ) ;
#8982=UNCERTAINTY_MEASURE_WITH_UNIT (LENGTH_MEASURE( 1.000000000000000082E-05 ), #9848, 'distance_accuracy_value', 'NONE');
#8993=CARTESIAN_POINT ( 'NONE',  ( 100.8561741729129153, 124.5000000010924737, -2.066987299999999195 ) ) ;
#9006=ORIENTED_EDGE ( 'NONE', *, *, #25843, .F. ) ;
#9012=CARTESIAN_POINT ( 'NONE',  ( 99.99999999999998579, 129.0000000000000000, 12.50000000000001066 ) ) ;
#9044=VECTOR ( 'NONE', #2550, 999.9999999999997726 ) ;
#9053=CARTESIAN_POINT ( 'NONE',  ( 99.99999999999998579, 124.1000000021849416, -2.499999999999997780 ) ) ;
#9065=CARTESIAN_POINT ( 'NONE',  ( 99.99999999999998579, 123.0000000000000000, -5.204170427930421283E-15 ) ) ;
#9092=DIRECTION ( 'NONE',  ( 8.659560562354927928E-17, -0.7071067811865482389, 0.7071067811865469066 ) ) ;
#9109=ORIENTED_EDGE ( 'NONE', *, *, #16138, .F. ) ;
#9132=CARTESIAN_POINT ( 'NONE',  ( 102.0669872999999797, 124.3500000010924822, -9.794112055954760458E-15 ) ) ;
#9144=CARTESIAN_POINT ( 'NONE',  ( 98.53841926354351699, 123.8500000010924680, -1.461580736456474794 ) ) ;
#9188=CARTESIAN_POINT ( 'NONE',  ( 101.4615807364564546, 124.0500000010924850, 1.461580736456455476 ) ) ;
#9190=CARTESIAN_POINT ( 'NONE',  ( 102.4999999999999858, 123.9000000021849530, -9.847140817659276890E-15 ) ) ;
#9204=DIRECTION ( 'NONE',  ( 0.000000000000000000, 1.000000000000000000, 0.000000000000000000 ) ) ;
#9209=CARTESIAN_POINT ( 'NONE',  ( 99.99999999999998579, 138.0000000000000000, -12.50000000000002132 ) ) ;
#9211=CARTESIAN_POINT ( 'NONE',  ( 99.99999999999998579, 138.0000000000000000, 12.50000000000001066 ) ) ;
#9230=FACE_OUTER_BOUND ( 'NONE', #964, .T. ) ;
#9232=CARTESIAN_POINT ( 'NONE',  ( 99.99999999999998579, 130.0000000000000000, -0.5000000000000138778 ) ) ;
#9248=CARTESIAN_POINT ( 'NONE',  ( 97.99846057881282491, 123.0000000000000142, -0.5333343844930795719 ) ) ;
#9253=CARTESIAN_POINT ( 'NONE',  ( 100.9550382616159538, 122.9999999999999716, 2.227387293901141430 ) ) ;
#9321=EDGE_CURVE ( 'NONE', #16572, #6030, #8219, .T. ) ;
#9339=EDGE_CURVE ( 'NONE', #11544, #20557, #18649, .T. ) ;
#9367=CARTESIAN_POINT ( 'NONE',  ( 99.14382582708707048, 123.9000000010924794, 2.066987299999979211 ) ) ;
#9452=CARTESIAN_POINT ( 'NONE',  ( 99.14382582708707048, 123.1000000010924822, 2.066987299999979211 ) ) ;
#9456=EDGE_LOOP ( 'NONE', ( #9109, #20168, #25538, #10951 ) ) ;
#9464=CARTESIAN_POINT ( 'NONE',  ( 98.53841926354351699, 123.6500000010924794, -1.461580736456474794 ) ) ;
#9471=DIRECTION ( 'NONE',  ( -0.000000000000000000, -1.000000000000000000, -0.000000000000000000 ) ) ;
#9512=CARTESIAN_POINT ( 'NONE',  ( 97.93301269999999192, 124.5000000010924879, -0.8561741729129505041 ) ) ;
#9530=CARTESIAN_POINT ( 'NONE',  ( 98.09035273295538104, 123.0000000000000142, 0.7910017786517971050 ) ) ;
#9543=VERTEX_POINT ( 'NONE', #6498 ) ;
#9586=ORIENTED_EDGE ( 'NONE', *, *, #17805, .F. ) ;
#9596=CARTESIAN_POINT ( 'NONE',  ( 101.4615807364564546, 122.6500000010924794, -1.461580736456474794 ) ) ;
#9618=( NAMED_UNIT ( * ) PLANE_ANGLE_UNIT ( ) SI_UNIT ( $, .RADIAN. ) );
#9650=CARTESIAN_POINT ( 'NONE',  ( 99.99999999999998579, 123.3000000021849587, -2.499999999999997780 ) ) ;
#9651=CARTESIAN_POINT ( 'NONE',  ( 97.93301269999999192, 123.8000000010924850, 0.8561741729129329626 ) ) ;
#9694=CARTESIAN_POINT ( 'NONE',  ( 99.99999999999998579, 129.0000000000000000, -5.204170427930421283E-15 ) ) ;
#9698=CARTESIAN_POINT ( 'NONE',  ( 101.7677669529663547, 124.5000000000000000, 1.767766952966350891 ) ) ;
#9711=DIRECTION ( 'NONE',  ( -0.000000000000000000, -1.000000000000000000, -0.000000000000000000 ) ) ;
#9722=CARTESIAN_POINT ( 'NONE',  ( 98.23223304703363112, 123.2999999999999972, -1.767766952966370209 ) ) ;
#9737=CARTESIAN_POINT ( 'NONE',  ( 97.93301269999999192, 123.7000000010924765, -0.8561741729129505041 ) ) ;
#9749=CARTESIAN_POINT ( 'NONE',  ( 100.8561741729129295, 124.3000000010924850, -2.066987299999998751 ) ) ;
#9758=SHAPE_REPRESENTATION_RELATIONSHIP ( 'NONE' , 'NONE' ,  #10045, #24660 ) ;
#9787=EDGE_CURVE ( 'NONE', #8172, #15313, #7659, .T. ) ;
#9808=( BOUNDED_CURVE ( )  B_SPLINE_CURVE ( 2, ( #24856, #496, #11719, #11437, #18009 ),
 .UNSPECIFIED., .F., .T. ) 
 B_SPLINE_CURVE_WITH_KNOTS ( ( 3, 2, 3 ),
 ( 0.000000000000000000, 0.04166666666666694885, 0.08333333333333389770 ),
 .UNSPECIFIED. ) 
 CURVE ( )  GEOMETRIC_REPRESENTATION_ITEM ( )  RATIONAL_B_SPLINE_CURVE ( ( 1.000000000000000000, 0.9238795325112867385, 1.000000000000000000, 0.9238795325112857393, 1.000000000000001110 ) ) 
 REPRESENTATION_ITEM ( '' )  );
#9818=EDGE_CURVE ( 'NONE', #22175, #18860, #23151, .T. ) ;
#9834=CARTESIAN_POINT ( 'NONE',  ( 98.23223304703363112, 123.5000000000000000, 1.767766952966351557 ) ) ;
#9848=( LENGTH_UNIT ( ) NAMED_UNIT ( * ) SI_UNIT ( .MILLI., .METRE. ) );
#9876=CARTESIAN_POINT ( 'NONE',  ( 101.4615807364564546, 124.2500000010924879, -1.461580736456474794 ) ) ;
#9916=DIRECTION ( 'NONE',  ( 0.000000000000000000, 0.000000000000000000, 1.000000000000000000 ) ) ;
#9922=CARTESIAN_POINT ( 'NONE',  ( 99.99999999999998579, 122.7500000010924879, -2.066987299999998751 ) ) ;
#9967=CARTESIAN_POINT ( 'NONE',  ( 102.4999999999999858, 123.7999999999999972, -9.847140817659276890E-15 ) ) ;
#9978=COLOUR_RGB ( '', 0.31764706, 0.68627451, 0.89019608) ;
#10010=CARTESIAN_POINT ( 'NONE',  ( 102.0669872999999939, 124.1000000010924964, 0.8561741729129311862 ) ) ;
#10020=FACE_OUTER_BOUND ( 'NONE', #27839, .T. ) ;
#10022=ORIENTED_EDGE ( 'NONE', *, *, #19598, .T. ) ;
#10045=SHAPE_REPRESENTATION ( 'Integrated Vacuum Pressure Gauge', ( #26844 ), #7245 ) ;
#10051=EDGE_CURVE ( 'NONE', #20981, #23148, #3444, .T. ) ;
#10054=CARTESIAN_POINT ( 'NONE',  ( 97.50000000000000000, 124.2500000021849758, -1.035533905932742416 ) ) ;
#10055=CARTESIAN_POINT ( 'NONE',  ( 99.99999999999998579, 128.0000000000000000, -5.204170427930421283E-15 ) ) ;
#10060=CARTESIAN_POINT ( 'NONE',  ( 99.99999999999998579, 123.3500000010924680, 2.066987299999980099 ) ) ;
#10097=CYLINDRICAL_SURFACE ( 'NONE', #15413, 12.50000000000001599 ) ;
#10099=CARTESIAN_POINT ( 'NONE',  ( 98.53841926354351699, 123.0500000010924850, -1.461580736456474794 ) ) ;
#10111=CARTESIAN_POINT ( 'NONE',  ( 99.99999999999998579, 124.1000000021849416, -2.499999999999997780 ) ) ;
#10148=CIRCLE ( 'NONE', #23386, 12.50000000000001599 ) ;
#10162=( LENGTH_UNIT ( ) NAMED_UNIT ( * ) SI_UNIT ( .MILLI., .METRE. ) );
#10191=CARTESIAN_POINT ( 'NONE',  ( 98.53841926354351699, 123.2500000010924737, 1.461580736456455920 ) ) ;
#10193=AXIS2_PLACEMENT_3D ( 'NONE', #27944, #23389, #17236 ) ;
#10235=CARTESIAN_POINT ( 'NONE',  ( 101.0355339059327378, 124.7500000000000142, -2.499999999999997780 ) ) ;
#10254=ORIENTED_EDGE ( 'NONE', *, *, #6847, .F. ) ;
#10297=CIRCLE ( 'NONE', #23091, 12.50000000000001599 ) ;
#10322=FACE_BOUND ( 'NONE', #24881, .T. ) ;
#10332=CARTESIAN_POINT ( 'NONE',  ( 99.99999999999998579, 122.9500000010924765, -2.066987299999998751 ) ) ;
#10362=ORIENTED_EDGE ( 'NONE', *, *, #22515, .F. ) ;
#10415=LINE ( 'NONE', #3879, #5499 ) ;
#10471=DIRECTION ( 'NONE',  ( -0.000000000000000000, -1.000000000000000000, -0.000000000000000000 ) ) ;
#10476=CARTESIAN_POINT ( 'NONE',  ( 98.53841926354351699, 123.8500000010924680, -1.461580736456474794 ) ) ;
#10481=FACE_OUTER_BOUND ( 'NONE', #20978, .T. ) ;
#10493=ORIENTED_EDGE ( 'NONE', *, *, #9321, .T. ) ;
#10518=CARTESIAN_POINT ( 'NONE',  ( 98.96446609406727646, 123.2500000000000000, -2.499999999999997780 ) ) ;
#10578=EDGE_LOOP ( 'NONE', ( #16832, #12852, #3728, #3271, #22365, #26400, #11510, #9586 ) ) ;
#10582=AXIS2_PLACEMENT_3D ( 'NONE', #12297, #20881, #3210 ) ;
#10598=CARTESIAN_POINT ( 'NONE',  ( 99.99999999999998579, 123.2000000000000028, -2.499999999999997780 ) ) ;
#10642=PRODUCT_DEFINITION ( 'UNKNOWN', '', #1314, #14319 ) ;
#10702=EDGE_LOOP ( 'NONE', ( #18144, #3624, #8878, #24353 ) ) ;
#10706=CARTESIAN_POINT ( 'NONE',  ( 101.7677669209684552, 123.0000000000000000, 1.767766984964258992 ) ) ;
#10722=CARTESIAN_POINT ( 'NONE',  ( 99.99999999999998579, 128.0000000000000000, -5.204170427930421283E-15 ) ) ;
#10768=APPLICATION_CONTEXT ( 'automotive_design' ) ;
#10840=CARTESIAN_POINT ( 'NONE',  ( 97.93301270000000613, 123.9000000010924794, -0.8561741729129506151 ) ) ;
#10911=DIRECTION ( 'NONE',  ( -0.000000000000000000, -1.000000000000000000, -0.000000000000000000 ) ) ;
#10914=VERTEX_POINT ( 'NONE', #18722 ) ;
#10941=CARTESIAN_POINT ( 'NONE',  ( 98.72729855789484077, 123.0000000000000568, -1.650814227560484460 ) ) ;
#10947=CONICAL_SURFACE ( 'NONE', #6801, 11.50000000000001776, 0.7853981633974473908 ) ;
#10951=ORIENTED_EDGE ( 'NONE', *, *, #3170, .F. ) ;
#10979=CARTESIAN_POINT ( 'NONE',  ( 99.99999999999998579, 124.1500000010924651, 2.066987299999980099 ) ) ;
#10988=ORIENTED_EDGE ( 'NONE', *, *, #21874, .T. ) ;
#11018=CIRCLE ( 'NONE', #10582, 2.500000000000008882 ) ;
#11130=AXIS2_PLACEMENT_3D ( 'NONE', #19028, #8060, #23186 ) ;
#11139=ORIENTED_EDGE ( 'NONE', *, *, #8072, .F. ) ;
#11168=DIRECTION ( 'NONE',  ( 0.000000000000000000, 0.000000000000000000, -1.000000000000000000 ) ) ;
#11170=CARTESIAN_POINT ( 'NONE',  ( 98.96446609406726225, 124.3500000000000085, 2.499999999999981348 ) ) ;
#11200=DIRECTION ( 'NONE',  ( 0.000000000000000000, 0.000000000000000000, -1.000000000000000000 ) ) ;
#11245=PRODUCT ( 'Integrated Vacuum Pressure Gauge', 'Integrated Vacuum Pressure Gauge', '', ( #25373 ) ) ;
#11342=STYLED_ITEM ( 'NONE', ( #748 ), #7835 ) ;
#11351=LINE ( 'NONE', #13344, #9044 ) ;
#11366=CARTESIAN_POINT ( 'NONE',  ( 98.95673454514873413, 123.0000000000000426, -1.805156233539860100 ) ) ;
#11422=ADVANCED_FACE ( 'NONE', ( #9230 ), #10947, .T. ) ;
#11437=CARTESIAN_POINT ( 'NONE',  ( 98.96446609406724804, 124.8499999999999943, -2.500000000000008438 ) ) ;
#11448=CARTESIAN_POINT ( 'NONE',  ( 99.14382582708708469, 123.1000000010924822, 2.066987299999979655 ) ) ;
#11495=CARTESIAN_POINT ( 'NONE',  ( 97.93301270000000613, 124.7500000010924737, -9.540979117872439019E-15 ) ) ;
#11510=ORIENTED_EDGE ( 'NONE', *, *, #8481, .T. ) ;
#11533=CARTESIAN_POINT ( 'NONE',  ( 98.53841926354351699, 124.6500000010924651, -1.461580736456474794 ) ) ;
#11544=VERTEX_POINT ( 'NONE', #9650 ) ;
#11575=CARTESIAN_POINT ( 'NONE',  ( 101.4615807364564546, 123.2500000010924879, 1.461580736456455476 ) ) ;
#11589=CARTESIAN_POINT ( 'NONE',  ( 102.0669873000000081, 123.4000000010924794, -0.8561741729129508371 ) ) ;
#11633=CARTESIAN_POINT ( 'NONE',  ( 99.14382582708707048, 124.4000000010924794, -2.066987299999999195 ) ) ;
#11687=SURFACE_SIDE_STYLE ('',( #2743 ) ) ;
#11688=AXIS2_PLACEMENT_3D ( 'NONE', #18403, #5721, #3578 ) ;
#11716=DIRECTION ( 'NONE',  ( -0.000000000000000000, -1.000000000000000000, -0.000000000000000000 ) ) ;
#11718=CARTESIAN_POINT ( 'NONE',  ( 99.99999999999998579, 122.7500000010924879, -2.066987299999998751 ) ) ;
#11719=CARTESIAN_POINT ( 'NONE',  ( 98.23223304703363112, 124.8999999999999915, -1.767766952966370209 ) ) ;
#11731=CARTESIAN_POINT ( 'NONE',  ( 100.8561741729129437, 124.0000000010925021, 2.066987299999979655 ) ) ;
#11778=CARTESIAN_POINT ( 'NONE',  ( 100.8561741729129153, 124.3000000010924708, -2.066987299999999195 ) ) ;
#11781=CARTESIAN_POINT ( 'NONE',  ( 101.7677669209684552, 123.0000000000000000, 1.767766984964258992 ) ) ;
#11822=CARTESIAN_POINT ( 'NONE',  ( 101.7677669529663547, 124.7000000000000028, -1.767766952966370209 ) ) ;
#11843=EDGE_LOOP ( 'NONE', ( #22158, #26767, #5447, #24228, #16169, #10493, #1628 ) ) ;
#11862=CARTESIAN_POINT ( 'NONE',  ( 98.53841926354351699, 123.6500000010924794, -1.461580736456474794 ) ) ;
#11899=CARTESIAN_POINT ( 'NONE',  ( 99.99999999999998579, 128.0000000000000000, 2.500000000000003553 ) ) ;
#11963=CARTESIAN_POINT ( 'NONE',  ( 97.50000000000000000, 124.1499999999999915, -1.035533905932742416 ) ) ;
#11971=LINE ( 'NONE', #25235, #25742 ) ;
#11990=AXIS2_PLACEMENT_3D ( 'NONE', #15878, #4786, #24302 ) ;
#12002=CARTESIAN_POINT ( 'NONE',  ( 99.14382582708707048, 122.8000000010924708, -2.066987299999999195 ) ) ;
#12052=CARTESIAN_POINT ( 'NONE',  ( 99.99999999999998579, 123.7500000010924737, -2.066987299999998751 ) ) ;
#12086=ORIENTED_EDGE ( 'NONE', *, *, #23440, .F. ) ;
#12094=CARTESIAN_POINT ( 'NONE',  ( 98.53841926354351699, 124.0500000010924708, 1.461580736456455920 ) ) ;
#12099=FACE_OUTER_BOUND ( 'NONE', #9456, .T. ) ;
#12111=ADVANCED_FACE ( 'NONE', ( #14994 ), #21724, .T. ) ;
#12138=CARTESIAN_POINT ( 'NONE',  ( 102.0669872999999797, 124.1500000010924794, -9.794112055954760458E-15 ) ) ;
#12141=DIRECTION ( 'NONE',  ( -0.000000000000000000, -1.000000000000000000, -0.000000000000000000 ) ) ;
#12164=FACE_OUTER_BOUND ( 'NONE', #25421, .T. ) ;
#12180=FACE_OUTER_BOUND ( 'NONE', #27704, .T. ) ;
#12182=CARTESIAN_POINT ( 'NONE',  ( 102.4999999999999858, 123.9000000021849530, -9.847140817659276890E-15 ) ) ;
#12189=CARTESIAN_POINT ( 'NONE',  ( 97.93301269999999192, 124.0000000010924879, 0.8561741729129329626 ) ) ;
#12217=AXIS2_PLACEMENT_3D ( 'NONE', #26346, #23505, #28200 ) ;
#12227=CARTESIAN_POINT ( 'NONE',  ( 98.96446609406724804, 123.6500000021849672, 2.499999999999969802 ) ) ;
#12230=CARTESIAN_POINT ( 'NONE',  ( 100.8561741729129153, 122.9000000010924936, -2.066987299999999195 ) ) ;
#12276=( BOUNDED_CURVE ( )  B_SPLINE_CURVE ( 2, ( #5065, #26588, #15873, #13439, #26731, #9749, #22166, #15734, #24868, #6903, #9188, #11731, #1081, #20309, #5349, #13729, #2785, #2644, #9464, #18459, #3066, #18167, #24438, #11589, #26879, #4925, #16013, #15591, #7324, #11448, #22451, #4779, #7176 ),
 .UNSPECIFIED., .F., .T. ) 
 B_SPLINE_CURVE_WITH_KNOTS ( ( 3, 2, 2, 2, 2, 2, 2, 2, 2, 2, 2, 2, 2, 2, 2, 2, 3 ),
 ( 0.000000000000000000, 0.04166666666666666435, 0.08333333333333332871, 0.1250000000000000000, 0.1666666666666666574, 0.2083333333333333426, 0.2500000000000000000, 0.2916666666666666852, 0.3333333333333333148, 0.3750000000000000000, 0.4166666666666666852, 0.4583333333333333148, 0.5000000000000000000, 0.5416666666666666297, 0.5833333333333333703, 0.6250000000000000000, 0.6458333337712076627 ),
 .UNSPECIFIED. ) 
 CURVE ( )  GEOMETRIC_REPRESENTATION_ITEM ( )  RATIONAL_B_SPLINE_CURVE ( ( 1.000000000000000000, 0.9238795325112867385, 1.000000000000000000, 0.9238795325112867385, 1.000000000000000000, 0.9238795325112867385, 1.000000000000000000, 0.9238795325112867385, 1.000000000000000000, 0.9238795325112867385, 1.000000000000000000, 0.9238795325112867385, 1.000000000000000000, 0.9238795325112867385, 1.000000000000000000, 0.9238795325112867385, 1.000000000000000000, 0.9238795325112867385, 1.000000000000000000, 0.9238795325112867385, 1.000000000000000000, 0.9238795325112867385, 1.000000000000000000, 0.9238795325112867385, 1.000000000000000000, 0.9238795325112867385, 1.000000000000000000, 0.9238795325112867385, 1.000000000000000000, 0.9238795325112867385, 1.000000000000000000, 0.9619397654556945954, 0.9619397662556433692 ) ) 
 REPRESENTATION_ITEM ( '' )  );
#12281=EDGE_CURVE ( 'NONE', #20557, #23148, #1296, .T. ) ;
#12297=CARTESIAN_POINT ( 'NONE',  ( 99.99999999999998579, 128.0000000000000000, -5.204170427930421283E-15 ) ) ;
#12316=UNCERTAINTY_MEASURE_WITH_UNIT (LENGTH_MEASURE( 1.000000000000000082E-05 ), #10162, 'distance_accuracy_value', 'NONE');
#12323=ADVANCED_FACE ( 'NONE', ( #1333 ), #27826, .T. ) ;
#12327=CARTESIAN_POINT ( 'NONE',  ( 102.4999999999999716, 123.8500000021849416, 1.035533905932722876 ) ) ;
#12336=CARTESIAN_POINT ( 'NONE',  ( 100.8561741729129295, 123.4000000010924794, 2.066987299999979211 ) ) ;
#12372=DIRECTION ( 'NONE',  ( -0.000000000000000000, -1.000000000000000000, -0.000000000000000000 ) ) ;
#12375=CARTESIAN_POINT ( 'NONE',  ( 102.0669872999999939, 122.8000000010924708, -0.8561741729129507261 ) ) ;
#12464=DIRECTION ( 'NONE',  ( 0.000000000000000000, 0.7071067811865469066, 0.7071067811865482389 ) ) ;
#12527=EDGE_CURVE ( 'NONE', #487, #16572, #10415, .T. ) ;
#12563=CARTESIAN_POINT ( 'NONE',  ( 99.99999999999998579, 128.0000000000000000, -5.204170427930421283E-15 ) ) ;
#12564=DIRECTION ( 'NONE',  ( 0.000000000000000000, 1.000000000000000000, 0.000000000000000000 ) ) ;
#12568=( BOUNDED_SURFACE ( )  B_SPLINE_SURFACE ( 1, 2, ( 
 ( #550, #9512, #7365, #11633, #2688, #11778, #22493, #1124, #26778, #20640, #16352, #2958, #694, #9367, #22782, #9651, #18062, #5249, #841, #18212, #16060, #24768, #7512, #25051, #16206, #13914, #17924, #22641, #3109, #24910, #5393, #14337, #3674, #1260, #14481, #25736, #9922, #3532, #12607, #22922, #25185 ),
 ( #8070, #21333, #21055, #18772, #3381, #8210, #18903, #5673, #18638, #16899, #6220, #1539, #20918, #25597, #27342, #12189, #16631, #1400, #10476, #27477, #12052, #7801, #5810, #17033, #27750, #23198, #6081, #12336, #10060, #3804, #10191, #27886, #27614, #7934, #19184, #25323, #10332, #14747, #16490, #23055, #1812 ) ),
 .UNSPECIFIED., .F., .F., .F. ) 
 B_SPLINE_SURFACE_WITH_KNOTS ( ( 2, 2 ),
 ( 3, 2, 2, 2, 2, 2, 2, 2, 2, 2, 2, 2, 2, 2, 2, 2, 2, 2, 2, 2, 3 ),
 ( 0.000000000000000000, 1.000000000000000000 ),
 ( 0.000000000000000000, 0.04166666666666666435, 0.08333333333333332871, 0.1250000000000000000, 0.1666666666666666574, 0.2083333333333333426, 0.2500000000000000000, 0.2916666666666666852, 0.3333333333333333148, 0.3750000000000000000, 0.4166666666666666852, 0.4583333333333333148, 0.5000000000000000000, 0.5416666666666666297, 0.5833333333333333703, 0.6250000000000000000, 0.6666666666666666297, 0.7083333333333333703, 0.7500000000000000000, 0.7916666666666666297, 0.8333333333333333703 ),
 .UNSPECIFIED. ) 
 GEOMETRIC_REPRESENTATION_ITEM ( )  RATIONAL_B_SPLINE_SURFACE ( (
 ( 1.000000000000000000, 0.9238795325112867385, 1.000000000000000000, 0.9238795325112867385, 1.000000000000000000, 0.9238795325112867385, 1.000000000000000000, 0.9238795325112867385, 1.000000000000000000, 0.9238795325112867385, 1.000000000000000000, 0.9238795325112867385, 1.000000000000000000, 0.9238795325112867385, 1.000000000000000000, 0.9238795325112867385, 1.000000000000000000, 0.9238795325112867385, 1.000000000000000000, 0.9238795325112867385, 1.000000000000000000, 0.9238795325112867385, 1.000000000000000000, 0.9238795325112867385, 1.000000000000000000, 0.9238795325112867385, 1.000000000000000000, 0.9238795325112867385, 1.000000000000000000, 0.9238795325112867385, 1.000000000000000000, 0.9238795325112867385, 1.000000000000000000, 0.9238795325112867385, 1.000000000000000000, 0.9238795325112867385, 1.000000000000000000, 0.9238795325112867385, 1.000000000000000000, 0.9238795325112867385, 1.000000000000000000),
 ( 1.000000000000000000, 0.9238795325112867385, 1.000000000000000000, 0.9238795325112867385, 1.000000000000000000, 0.9238795325112867385, 1.000000000000000000, 0.9238795325112867385, 1.000000000000000000, 0.9238795325112867385, 1.000000000000000000, 0.9238795325112867385, 1.000000000000000000, 0.9238795325112867385, 1.000000000000000000, 0.9238795325112867385, 1.000000000000000000, 0.9238795325112867385, 1.000000000000000000, 0.9238795325112867385, 1.000000000000000000, 0.9238795325112867385, 1.000000000000000000, 0.9238795325112867385, 1.000000000000000000, 0.9238795325112867385, 1.000000000000000000, 0.9238795325112867385, 1.000000000000000000, 0.9238795325112867385, 1.000000000000000000, 0.9238795325112867385, 1.000000000000000000, 0.9238795325112867385, 1.000000000000000000, 0.9238795325112867385, 1.000000000000000000, 0.9238795325112867385, 1.000000000000000000, 0.9238795325112867385, 1.000000000000000000) ) ) 
 REPRESENTATION_ITEM ( '' )  SURFACE ( )  );
#12576=DIRECTION ( 'NONE',  ( 0.000000000000000000, 0.000000000000000000, 1.000000000000000000 ) ) ;
#12586=UNCERTAINTY_MEASURE_WITH_UNIT (LENGTH_MEASURE( 1.000000000000000082E-05 ), #16738, 'distance_accuracy_value', 'NONE');
#12607=CARTESIAN_POINT ( 'NONE',  ( 101.4615807364564546, 122.6500000010924794, -1.461580736456474794 ) ) ;
#12663=AXIS2_PLACEMENT_3D ( 'NONE', #20998, #26607, #17760 ) ;
#12743=FACE_OUTER_BOUND ( 'NONE', #6299, .T. ) ;
#12748=CARTESIAN_POINT ( 'NONE',  ( 99.99999999999998579, 124.0000000000000000, -2.499999999999997780 ) ) ;
#12792=EDGE_CURVE ( 'NONE', #25689, #14731, #17776, .T. ) ;
#12836=CARTESIAN_POINT ( 'NONE',  ( 101.7677669209684552, 123.0000000000000000, 1.767766984964258992 ) ) ;
#12837=CARTESIAN_POINT ( 'NONE',  ( 99.92084351319844870, 123.0000000000000142, -2.153125375274123510 ) ) ;
#12852=ORIENTED_EDGE ( 'NONE', *, *, #21874, .F. ) ;
#12855=CARTESIAN_POINT ( 'NONE',  ( 102.4999999999999858, 124.5500000000000256, 1.035533905932722876 ) ) ;
#12915=ADVANCED_FACE ( 'NONE', ( #22393 ), #13828, .T. ) ;
#12921=CARTESIAN_POINT ( 'NONE',  ( 102.4999999999999716, 123.0500000000000114, -1.035533905932742638 ) ) ;
#12970=CARTESIAN_POINT ( 'NONE',  ( 98.82914575430085335, 123.0259891538152743, -1.752307227213801832 ) ) ;
#13039=DIRECTION ( 'NONE',  ( -0.000000000000000000, -1.000000000000000000, -0.000000000000000000 ) ) ;
#13107=CARTESIAN_POINT ( 'NONE',  ( 100.8561741729129295, 124.5000000010924737, -2.066987299999998751 ) ) ;
#13180=VERTEX_POINT ( 'NONE', #707 ) ;
#13199=VERTEX_POINT ( 'NONE', #2704 ) ;
#13276=CARTESIAN_POINT ( 'NONE',  ( 101.0355339059327378, 124.7500000000000284, -2.499999999999988010 ) ) ;
#13328=ORIENTED_EDGE ( 'NONE', *, *, #23943, .T. ) ;
#13344=CARTESIAN_POINT ( 'NONE',  ( 97.71650635000000307, 124.8750000005462368, -9.540979117872439019E-15 ) ) ;
#13406=VECTOR ( 'NONE', #8063, 1000.000000000000000 ) ;
#13424=ORIENTED_EDGE ( 'NONE', *, *, #17353, .F. ) ;
#13439=CARTESIAN_POINT ( 'NONE',  ( 99.14382582708708469, 124.4000000010924794, -2.066987299999998751 ) ) ;
#13445=FACE_OUTER_BOUND ( 'NONE', #19144, .T. ) ;
#13520=AXIS2_PLACEMENT_3D ( 'NONE', #13521, #2436, #22379 ) ;
#13521=CARTESIAN_POINT ( 'NONE',  ( 99.99999999999998579, 130.0000000000000000, -5.204170427930421283E-15 ) ) ;
#13545=EDGE_LOOP ( 'NONE', ( #8353, #24432, #2068, #26910 ) ) ;
#13546=CARTESIAN_POINT ( 'NONE',  ( 97.93301270000000613, 123.2000000010924765, 0.8561741729129328515 ) ) ;
#13553=ORIENTED_EDGE ( 'NONE', *, *, #9339, .F. ) ;
#13578=VERTEX_POINT ( 'NONE', #23757 ) ;
#13634=CARTESIAN_POINT ( 'NONE',  ( 99.99999999999998579, 138.0000000000000000, 11.50000000000001243 ) ) ;
#13635=ORIENTED_EDGE ( 'NONE', *, *, #9787, .F. ) ;
#13717=CARTESIAN_POINT ( 'NONE',  ( 102.0669872999999939, 123.4000000010924936, -0.8561741729129507261 ) ) ;
#13729=CARTESIAN_POINT ( 'NONE',  ( 97.93301270000000613, 123.8000000010924566, 0.8561741729129328515 ) ) ;
#13770=AXIS2_PLACEMENT_3D ( 'NONE', #20482, #24892, #5089 ) ;
#13774=CARTESIAN_POINT ( 'NONE',  ( 99.99999999999998579, 123.3000000021849587, -2.499999999999997780 ) ) ;
#13786=( BOUNDED_CURVE ( )  B_SPLINE_CURVE ( 2, ( #21805, #24218, #21661, #4270, #2138, #4026, #4552, #6960, #22227 ),
 .UNSPECIFIED., .F., .F. ) 
 B_SPLINE_CURVE_WITH_KNOTS ( ( 3, 2, 2, 2, 3 ),
 ( 0.4166666666666667407, 0.4583333333333334259, 0.5000000000000002220, 0.5416666666666668517, 0.5833333333333337034 ),
 .UNSPECIFIED. ) 
 CURVE ( )  GEOMETRIC_REPRESENTATION_ITEM ( )  RATIONAL_B_SPLINE_CURVE ( ( 0.9999999999999998890, 0.9238795325112868495, 1.000000000000000000, 0.9238795325112867385, 1.000000000000000000, 0.9238795325112867385, 1.000000000000000000, 0.9238795325112861834, 1.000000000000000666 ) ) 
 REPRESENTATION_ITEM ( '' )  );
#13825=DIRECTION ( 'NONE',  ( -0.000000000000000000, -1.000000000000000000, -0.000000000000000000 ) ) ;
#13828=( BOUNDED_SURFACE ( )  B_SPLINE_SURFACE ( 1, 2, ( 
 ( #308, #449, #11533, #4724, #24673, #8993, #22112, #26389, #9132, #17825, #26530, #15681, #14244, #25370, #12094, #18680, #16103, #18811, #22825, #18945, #24809, #5579, #20821, #5436, #7556, #27518, #14521, #18541, #5850, #22965, #7841, #1028, #22683, #23236, #10099, #5716, #3713, #12230, #27245, #12375, #3153 ),
 ( #5292, #27105, #16394, #13956, #7701, #10235, #11822, #16251, #21093, #7409, #9698, #20958, #1582, #1299, #20545, #3427, #3293, #11963, #25092, #14382, #18398, #24949, #1441, #14103, #9967, #23098, #27382, #16535, #20685, #1168, #9834, #25227, #3574, #7974, #16673, #10518, #21796, #4260, #27927, #12921, #17073 ) ),
 .UNSPECIFIED., .F., .F., .F. ) 
 B_SPLINE_SURFACE_WITH_KNOTS ( ( 2, 2 ),
 ( 3, 2, 2, 2, 2, 2, 2, 2, 2, 2, 2, 2, 2, 2, 2, 2, 2, 2, 2, 2, 3 ),
 ( 0.000000000000000000, 1.000000000000000000 ),
 ( 0.000000000000000000, 0.04166666666666666435, 0.08333333333333332871, 0.1250000000000000000, 0.1666666666666666574, 0.2083333333333333426, 0.2500000000000000000, 0.2916666666666666852, 0.3333333333333333148, 0.3750000000000000000, 0.4166666666666666852, 0.4583333333333333148, 0.5000000000000000000, 0.5416666666666666297, 0.5833333333333333703, 0.6250000000000000000, 0.6666666666666666297, 0.7083333333333333703, 0.7500000000000000000, 0.7916666666666666297, 0.8333333333333333703 ),
 .UNSPECIFIED. ) 
 GEOMETRIC_REPRESENTATION_ITEM ( )  RATIONAL_B_SPLINE_SURFACE ( (
 ( 1.000000000000000000, 0.9238795325112867385, 1.000000000000000000, 0.9238795325112867385, 1.000000000000000000, 0.9238795325112867385, 1.000000000000000000, 0.9238795325112867385, 1.000000000000000000, 0.9238795325112867385, 1.000000000000000000, 0.9238795325112867385, 1.000000000000000000, 0.9238795325112867385, 1.000000000000000000, 0.9238795325112867385, 1.000000000000000000, 0.9238795325112867385, 1.000000000000000000, 0.9238795325112867385, 1.000000000000000000, 0.9238795325112867385, 1.000000000000000000, 0.9238795325112867385, 1.000000000000000000, 0.9238795325112867385, 1.000000000000000000, 0.9238795325112867385, 1.000000000000000000, 0.9238795325112867385, 1.000000000000000000, 0.9238795325112867385, 1.000000000000000000, 0.9238795325112867385, 1.000000000000000000, 0.9238795325112867385, 1.000000000000000000, 0.9238795325112867385, 1.000000000000000000, 0.9238795325112867385, 1.000000000000000000),
 ( 1.000000000000000000, 0.9238795325112867385, 1.000000000000000000, 0.9238795325112867385, 1.000000000000000000, 0.9238795325112867385, 1.000000000000000000, 0.9238795325112867385, 1.000000000000000000, 0.9238795325112867385, 1.000000000000000000, 0.9238795325112867385, 1.000000000000000000, 0.9238795325112867385, 1.000000000000000000, 0.9238795325112867385, 1.000000000000000000, 0.9238795325112867385, 1.000000000000000000, 0.9238795325112867385, 1.000000000000000000, 0.9238795325112867385, 1.000000000000000000, 0.9238795325112867385, 1.000000000000000000, 0.9238795325112867385, 1.000000000000000000, 0.9238795325112867385, 1.000000000000000000, 0.9238795325112867385, 1.000000000000000000, 0.9238795325112867385, 1.000000000000000000, 0.9238795325112867385, 1.000000000000000000, 0.9238795325112867385, 1.000000000000000000, 0.9238795325112867385, 1.000000000000000000, 0.9238795325112867385, 1.000000000000000000) ) ) 
 REPRESENTATION_ITEM ( '' )  SURFACE ( )  );
#13857=CARTESIAN_POINT ( 'NONE',  ( 101.0355339059327378, 122.9500000021849502, 2.499999999999977796 ) ) ;
#13862=AXIS2_PLACEMENT_3D ( 'NONE', #6936, #2401, #11200 ) ;
#13880=ORIENTED_EDGE ( 'NONE', *, *, #5505, .T. ) ;
#13914=CARTESIAN_POINT ( 'NONE',  ( 102.0669872999999939, 123.3000000010924850, 0.8561741729129311862 ) ) ;
#13952=DIRECTION ( 'NONE',  ( -0.000000000000000000, 1.000000000000000000, -0.000000000000000000 ) ) ;
#13956=CARTESIAN_POINT ( 'NONE',  ( 98.96446609406727646, 124.8500000000000085, -2.499999999999997780 ) ) ;
#14002=CARTESIAN_POINT ( 'NONE',  ( 98.96446609406727646, 123.3500000021849701, -2.499999999999997780 ) ) ;
#14084=MECHANICAL_DESIGN_GEOMETRIC_PRESENTATION_REPRESENTATION('',(#18176),#22749);
#14088=AXIS2_PLACEMENT_3D ( 'NONE', #15971, #13825, #22549 ) ;
#14103=CARTESIAN_POINT ( 'NONE',  ( 102.4999999999999716, 123.8500000000000085, -1.035533905932742638 ) ) ;
#14115=LINE ( 'NONE', #24821, #17730 ) ;
#14142=CARTESIAN_POINT ( 'NONE',  ( 99.99999999999998579, 128.0000000000000000, -5.204170427930421283E-15 ) ) ;
#14145=CARTESIAN_POINT ( 'NONE',  ( 98.53841926354351699, 123.0500000010924850, 1.461580736456455920 ) ) ;
#14234=ORIENTED_EDGE ( 'NONE', *, *, #9321, .F. ) ;
#14244=CARTESIAN_POINT ( 'NONE',  ( 99.99999999999998579, 124.1500000010924651, 2.066987299999980099 ) ) ;
#14273=CARTESIAN_POINT ( 'NONE',  ( 102.4999999999999858, 123.0000000000000000, -8.724596124144689908E-15 ) ) ;
#14279=DIRECTION ( 'NONE',  ( 0.000000000000000000, 0.000000000000000000, 1.000000000000000000 ) ) ;
#14285=CARTESIAN_POINT ( 'NONE',  ( 97.93301270000000613, 124.5500000010924850, -9.540979117872439019E-15 ) ) ;
#14289=DIRECTION ( 'NONE',  ( 0.000000000000000000, 0.000000000000000000, 1.000000000000000000 ) ) ;
#14319=PRODUCT_DEFINITION_CONTEXT ( 'detailed design', #22453, 'design' ) ;
#14327=PLANE ( 'NONE',  #24336 ) ;
#14329=CARTESIAN_POINT ( 'NONE',  ( 97.50000000000000000, 123.4500000021849502, -1.035533905932742416 ) ) ;
#14334=LINE ( 'NONE', #7509, #27272 ) ;
#14337=CARTESIAN_POINT ( 'NONE',  ( 97.93301269999999192, 123.0000000010925163, 0.8561741729129329626 ) ) ;
#14382=CARTESIAN_POINT ( 'NONE',  ( 98.96446609406727646, 124.0499999999999972, -2.499999999999997780 ) ) ;
#14468=DIRECTION ( 'NONE',  ( 0.000000000000000000, -0.000000000000000000, 1.000000000000000000 ) ) ;
#14471=CARTESIAN_POINT ( 'NONE',  ( 101.0355339059327378, 123.7500000021849615, 2.499999999999977796 ) ) ;
#14481=CARTESIAN_POINT ( 'NONE',  ( 98.53841926354351699, 122.8500000010924680, -1.461580736456474794 ) ) ;
#14508=ORIENTED_EDGE ( 'NONE', *, *, #18939, .T. ) ;
#14521=CARTESIAN_POINT ( 'NONE',  ( 101.4615807364564546, 123.4500000010924765, 1.461580736456455476 ) ) ;
#14537=CARTESIAN_POINT ( 'NONE',  ( 98.23223304703363112, 124.2000000021849502, -1.767766952966370209 ) ) ;
#14629=CARTESIAN_POINT ( 'NONE',  ( 102.1844659708856540, 123.0000000000000284, 1.259047450927248235 ) ) ;
#14683=CARTESIAN_POINT ( 'NONE',  ( 99.99999999999998579, 129.0000000000000000, -5.204170427930421283E-15 ) ) ;
#14701=CARTESIAN_POINT ( 'NONE',  ( 100.6702820041304136, 123.0000000000000142, -2.125135801581156336 ) ) ;
#14713=EDGE_CURVE ( 'NONE', #17592, #1875, #3137, .T. ) ;
#14731=VERTEX_POINT ( 'NONE', #24368 ) ;
#14747=CARTESIAN_POINT ( 'NONE',  ( 100.8561741729129153, 122.9000000010924936, -2.066987299999999195 ) ) ;
#14768=ORIENTED_EDGE ( 'NONE', *, *, #8072, .T. ) ;
#14916=VECTOR ( 'NONE', #18915, 999.9999999999997726 ) ;
#14979=CARTESIAN_POINT ( 'NONE',  ( 100.5910519820011473, 122.9999999999999432, 2.314246848314063243 ) ) ;
#14994=FACE_OUTER_BOUND ( 'NONE', #13545, .T. ) ;
#15019=( BOUNDED_SURFACE ( )  B_SPLINE_SURFACE ( 1, 2, ( 
 ( #16480, #10054, #7926, #27604, #27469, #3523, #16623, #25315, #12182, #12327, #7794, #14471, #23189, #25177, #3665, #21048, #5665, #14329, #23001, #14002, #7744, #18445, #7604, #24855, #1068, #3471, #20726, #13857, #20863, #18298, #16293, #16574, #1345, #18582, #27286, #16001, #22725, #16432, #26866, #3191, #20585 ),
 ( #14285, #7312, #1210, #25130, #24715, #5617, #9876, #5335, #12138, #10010, #20444, #24996, #18720, #5193, #5475, #27418, #7881, #9737, #11862, #2906, #5052, #20295, #27152, #13717, #22439, #3332, #11575, #782, #16147, #9452, #14145, #3051, #18152, #22864, #22582, #12002, #11718, #925, #9596, #27006, #7453 ) ),
 .UNSPECIFIED., .F., .F., .T. ) 
 B_SPLINE_SURFACE_WITH_KNOTS ( ( 2, 2 ),
 ( 3, 2, 2, 2, 2, 2, 2, 2, 2, 2, 2, 2, 2, 2, 2, 2, 2, 2, 2, 2, 3 ),
 ( 0.000000000000000000, 1.000000000000000000 ),
 ( 0.000000000000000000, 0.04166666666666666435, 0.08333333333333332871, 0.1250000000000000000, 0.1666666666666666574, 0.2083333333333333426, 0.2500000000000000000, 0.2916666666666666852, 0.3333333333333333148, 0.3750000000000000000, 0.4166666666666666852, 0.4583333333333333148, 0.5000000000000000000, 0.5416666666666666297, 0.5833333333333333703, 0.6250000000000000000, 0.6666666666666666297, 0.7083333333333333703, 0.7500000000000000000, 0.7916666666666666297, 0.8333333333333333703 ),
 .UNSPECIFIED. ) 
 GEOMETRIC_REPRESENTATION_ITEM ( )  RATIONAL_B_SPLINE_SURFACE ( (
 ( 1.000000000000000000, 0.9238795325112867385, 1.000000000000000000, 0.9238795325112867385, 1.000000000000000000, 0.9238795325112867385, 1.000000000000000000, 0.9238795325112867385, 1.000000000000000000, 0.9238795325112867385, 1.000000000000000000, 0.9238795325112867385, 1.000000000000000000, 0.9238795325112867385, 1.000000000000000000, 0.9238795325112867385, 1.000000000000000000, 0.9238795325112867385, 1.000000000000000000, 0.9238795325112867385, 1.000000000000000000, 0.9238795325112867385, 1.000000000000000000, 0.9238795325112867385, 1.000000000000000000, 0.9238795325112867385, 1.000000000000000000, 0.9238795325112867385, 1.000000000000000000, 0.9238795325112867385, 1.000000000000000000, 0.9238795325112867385, 1.000000000000000000, 0.9238795325112867385, 1.000000000000000000, 0.9238795325112867385, 1.000000000000000000, 0.9238795325112867385, 1.000000000000000000, 0.9238795325112867385, 1.000000000000000000),
 ( 1.000000000000000000, 0.9238795325112867385, 1.000000000000000000, 0.9238795325112867385, 1.000000000000000000, 0.9238795325112867385, 1.000000000000000000, 0.9238795325112867385, 1.000000000000000000, 0.9238795325112867385, 1.000000000000000000, 0.9238795325112867385, 1.000000000000000000, 0.9238795325112867385, 1.000000000000000000, 0.9238795325112867385, 1.000000000000000000, 0.9238795325112867385, 1.000000000000000000, 0.9238795325112867385, 1.000000000000000000, 0.9238795325112867385, 1.000000000000000000, 0.9238795325112867385, 1.000000000000000000, 0.9238795325112867385, 1.000000000000000000, 0.9238795325112867385, 1.000000000000000000, 0.9238795325112867385, 1.000000000000000000, 0.9238795325112867385, 1.000000000000000000, 0.9238795325112867385, 1.000000000000000000, 0.9238795325112867385, 1.000000000000000000, 0.9238795325112867385, 1.000000000000000000, 0.9238795325112867385, 1.000000000000000000) ) ) 
 REPRESENTATION_ITEM ( '' )  SURFACE ( )  );
#15114=CARTESIAN_POINT ( 'NONE',  ( 99.29898749929290602, 122.9999999999999858, 2.154550021601044030 ) ) ;
#15125=VECTOR ( 'NONE', #10911, 1000.000000000000000 ) ;
#15165=B_SPLINE_CURVE_WITH_KNOTS ( 'NONE', 3,
 ( #18854, #27562, #8023, #16722, #5901, #1625, #25556, #27702, #6035, #8165, #23420, #14701, #3893, #4175, #12837, #6576, #17701, #8720 ),
 .UNSPECIFIED., .F., .F.,
 ( 4, 2, 2, 2, 2, 2, 2, 2, 4 ),
 ( 0.000000000000000000, 0.0005599264814053035114, 0.001119852962810607023, 0.001679779444215910534, 0.002239705925621214046, 0.002799632407026517340, 0.003359558888431821069, 0.003919485369837124797, 0.004479411851242428091 ),
 .UNSPECIFIED. ) ;
#15188=( BOUNDED_CURVE ( )  B_SPLINE_CURVE ( 2, ( #1315, #27668, #14537, #21248, #10111 ),
 .UNSPECIFIED., .F., .T. ) 
 B_SPLINE_CURVE_WITH_KNOTS ( ( 3, 2, 3 ),
 ( 0.000000000000000000, 0.04166666666666653945, 0.08333333333333307891 ),
 .UNSPECIFIED. ) 
 CURVE ( )  GEOMETRIC_REPRESENTATION_ITEM ( )  RATIONAL_B_SPLINE_CURVE ( ( 1.000000000000000000, 0.9238795325112867385, 1.000000000000000000, 0.9238795325112871826, 0.9999999999999995559 ) ) 
 REPRESENTATION_ITEM ( '' )  );
#15195=EDGE_CURVE ( 'NONE', #23831, #13180, #25010, .T. ) ;
#15257=CARTESIAN_POINT ( 'NONE',  ( 99.14382582708708469, 123.3000000010924708, 2.066987299999979655 ) ) ;
#15313=VERTEX_POINT ( 'NONE', #22879 ) ;
#15315=ORIENTED_EDGE ( 'NONE', *, *, #20663, .T. ) ;
#15337=CARTESIAN_POINT ( 'NONE',  ( 99.99999999999998579, 137.0000000000000000, -5.204170427930421283E-15 ) ) ;
#15413=AXIS2_PLACEMENT_3D ( 'NONE', #21229, #12372, #1713 ) ;
#15420=DIRECTION ( 'NONE',  ( 0.000000000000000000, 0.000000000000000000, -1.000000000000000000 ) ) ;
#15488=VERTEX_POINT ( 'NONE', #15982 ) ;
#15546=CARTESIAN_POINT ( 'NONE',  ( 97.93301270000000613, 123.1000000010924822, -0.8561741729129506151 ) ) ;
#15591=CARTESIAN_POINT ( 'NONE',  ( 100.8561741729129437, 123.2000000010924765, 2.066987299999979655 ) ) ;
#15657=EDGE_CURVE ( 'NONE', #18860, #20976, #14334, .T. ) ;
#15681=CARTESIAN_POINT ( 'NONE',  ( 100.8561741729129295, 124.2000000010924907, 2.066987299999979211 ) ) ;
#15721=CIRCLE ( 'NONE', #7073, 0.5000000000000086597 ) ;
#15734=CARTESIAN_POINT ( 'NONE',  ( 102.0669873000000081, 124.2000000010924623, -0.8561741729129508371 ) ) ;
#15750=EDGE_CURVE ( 'NONE', #13180, #11544, #2616, .T. ) ;
#15786=VECTOR ( 'NONE', #12141, 1000.000000000000000 ) ;
#15801=CARTESIAN_POINT ( 'NONE',  ( 99.99999999999998579, 129.0000000000000000, -12.50000000000002132 ) ) ;
#15836=ORIENTED_EDGE ( 'NONE', *, *, #4279, .T. ) ;
#15873=CARTESIAN_POINT ( 'NONE',  ( 98.53841926354351699, 124.4500000010924765, -1.461580736456474794 ) ) ;
#15878=CARTESIAN_POINT ( 'NONE',  ( 99.99999999999998579, 138.0000000000000000, -5.204170427930421283E-15 ) ) ;
#15913=LINE ( 'NONE', #13634, #26447 ) ;
#15971=CARTESIAN_POINT ( 'NONE',  ( 99.99999999999998579, 138.0000000000000000, -5.204170427930421283E-15 ) ) ;
#15982=CARTESIAN_POINT ( 'NONE',  ( 99.99999999999998579, 124.0000000000000000, -2.499999999999997780 ) ) ;
#16001=CARTESIAN_POINT ( 'NONE',  ( 98.96446609406727646, 122.5500000021849587, -2.499999999999997780 ) ) ;
#16013=CARTESIAN_POINT ( 'NONE',  ( 101.4615807364564546, 123.2500000010924879, 1.461580736456455476 ) ) ;
#16060=CARTESIAN_POINT ( 'NONE',  ( 99.99999999999998579, 123.5500000010924850, -2.066987299999998751 ) ) ;
#16075=CARTESIAN_POINT ( 'NONE',  ( 97.98586169945060931, 123.0000000000000568, 0.5387381024522378548 ) ) ;
#16103=CARTESIAN_POINT ( 'NONE',  ( 97.93301270000000613, 123.9500000010924765, -9.540979117872439019E-15 ) ) ;
#16138=EDGE_CURVE ( 'NONE', #14731, #4566, #15913, .T. ) ;
#16147=CARTESIAN_POINT ( 'NONE',  ( 99.99999999999998579, 123.1500000010924794, 2.066987299999980099 ) ) ;
#16152=AXIS2_PLACEMENT_3D ( 'NONE', #15337, #2260, #4527 ) ;
#16169=ORIENTED_EDGE ( 'NONE', *, *, #3840, .F. ) ;
#16206=CARTESIAN_POINT ( 'NONE',  ( 102.0669872999999797, 123.3500000010924680, -9.794112055954760458E-15 ) ) ;
#16251=CARTESIAN_POINT ( 'NONE',  ( 102.4999999999999716, 124.6500000000000199, -1.035533905932742638 ) ) ;
#16293=CARTESIAN_POINT ( 'NONE',  ( 98.23223304703363112, 122.8000000021849587, 1.767766952966351557 ) ) ;
#16352=CARTESIAN_POINT ( 'NONE',  ( 101.4615807364564546, 124.0500000010924850, 1.461580736456455476 ) ) ;
#16390=CARTESIAN_POINT ( 'NONE',  ( 97.50000000000000000, 123.5500000021849587, 1.035533905932725096 ) ) ;
#16394=CARTESIAN_POINT ( 'NONE',  ( 98.23223304703363112, 124.8999999999999915, -1.767766952966370209 ) ) ;
#16432=CARTESIAN_POINT ( 'NONE',  ( 101.0355339059327378, 122.4500000021849502, -2.499999999999997780 ) ) ;
#16480=CARTESIAN_POINT ( 'NONE',  ( 97.50000000000000000, 124.3000000021849587, -9.540979117872439019E-15 ) ) ;
#16490=CARTESIAN_POINT ( 'NONE',  ( 101.4615807364564546, 122.8500000010924680, -1.461580736456474794 ) ) ;
#16511=CARTESIAN_POINT ( 'NONE',  ( 101.7677669209684552, 123.0000000000000000, 1.767766984964258992 ) ) ;
#16532=CARTESIAN_POINT ( 'NONE',  ( 98.23223304703363112, 123.4000000021849530, -1.767766952966370209 ) ) ;
#16535=CARTESIAN_POINT ( 'NONE',  ( 101.0355339059327378, 123.6500000000000199, 2.499999999999977796 ) ) ;
#16572=VERTEX_POINT ( 'NONE', #23010 ) ;
#16574=CARTESIAN_POINT ( 'NONE',  ( 97.50000000000000000, 122.7500000021849615, 1.035533905932725096 ) ) ;
#16584=DIRECTION ( 'NONE',  ( -0.000000000000000000, -1.000000000000000000, -0.000000000000000000 ) ) ;
#16603=DIRECTION ( 'NONE',  ( 0.000000000000000000, 1.000000000000000000, 0.000000000000000000 ) ) ;
#16611=EDGE_LOOP ( 'NONE', ( #10022, #904, #22606, #6551 ) ) ;
#16618=ADVANCED_FACE ( 'NONE', ( #10020 ), #18728, .T. ) ;
#16620=ADVANCED_FACE ( 'NONE', ( #5765 ), #3626, .F. ) ;
#16623=CARTESIAN_POINT ( 'NONE',  ( 101.7677669529663547, 124.0000000021849615, -1.767766952966370209 ) ) ;
#16631=CARTESIAN_POINT ( 'NONE',  ( 97.93301270000000613, 123.9500000010924765, -9.540979117872439019E-15 ) ) ;
#16642=DIRECTION ( 'NONE',  ( -0.000000000000000000, -1.000000000000000000, -0.000000000000000000 ) ) ;
#16673=CARTESIAN_POINT ( 'NONE',  ( 98.23223304703363112, 123.2999999999999972, -1.767766952966370209 ) ) ;
#16706=DIRECTION ( 'NONE',  ( -0.000000000000000000, 1.000000000000000000, -0.000000000000000000 ) ) ;
#16722=CARTESIAN_POINT ( 'NONE',  ( 102.3302406096647843, 122.9999999999999289, -0.7272111440987778508 ) ) ;
#16738=( LENGTH_UNIT ( ) NAMED_UNIT ( * ) SI_UNIT ( .MILLI., .METRE. ) );
#16802=CARTESIAN_POINT ( 'NONE',  ( 99.99999999999998579, 129.0000000000000000, -5.204170427930421283E-15 ) ) ;
#16832=ORIENTED_EDGE ( 'NONE', *, *, #5505, .F. ) ;
#16852=ORIENTED_EDGE ( 'NONE', *, *, #18362, .F. ) ;
#16859=ORIENTED_EDGE ( 'NONE', *, *, #9818, .F. ) ;
#16899=CARTESIAN_POINT ( 'NONE',  ( 102.0669872999999939, 124.3000000010924566, 0.8561741729129311862 ) ) ;
#16984=ORIENTED_EDGE ( 'NONE', *, *, #17353, .T. ) ;
#17033=CARTESIAN_POINT ( 'NONE',  ( 102.0669872999999939, 123.6000000010924680, -0.8561741729129507261 ) ) ;
#17038=CARTESIAN_POINT ( 'NONE',  ( 99.99999999999998579, 128.0000000000000000, -5.204170427930421283E-15 ) ) ;
#17073=CARTESIAN_POINT ( 'NONE',  ( 102.4999999999999858, 123.0000000000000000, -9.847140817659276890E-15 ) ) ;
#17084=CARTESIAN_POINT ( 'NONE',  ( 97.93301270000000613, 124.6500000010924651, -9.540979117872439019E-15 ) ) ;
#17126=CARTESIAN_POINT ( 'NONE',  ( 98.81505309850513186, 123.0000000000000426, 1.864324913875618162 ) ) ;
#17157=CARTESIAN_POINT ( 'NONE',  ( 99.99999999999998579, 128.0000000000000000, 2.500000000000003553 ) ) ;
#17161=B_SPLINE_CURVE_WITH_KNOTS ( 'NONE', 3,
 ( #6443, #7103, #6965, #1904, #4848, #17126, #8297, #15114, #23834, #19412, #19135, #2711, #14979, #9253, #6303, #572, #24505, #10706 ),
 .UNSPECIFIED., .F., .F.,
 ( 4, 2, 2, 2, 2, 2, 2, 2, 4 ),
 ( 0.000000000000000000, 0.0005608035638250541540, 0.001121607127650108308, 0.001682410691475162787, 0.002243214255300217484, 0.002804017819125271746, 0.003364821382950326442, 0.003925624946775381138, 0.004486428510600435834 ),
 .UNSPECIFIED. ) ;
#17206=VECTOR ( 'NONE', #16642, 1000.000000000000000 ) ;
#17236=DIRECTION ( 'NONE',  ( 0.000000000000000000, 0.000000000000000000, -1.000000000000000000 ) ) ;
#17268=CARTESIAN_POINT ( 'NONE',  ( 97.93301270000000613, 123.9500000010924765, -9.540979117872439019E-15 ) ) ;
#17270=DIRECTION ( 'NONE',  ( 0.000000000000000000, -1.000000000000000000, 0.000000000000000000 ) ) ;
#17353=EDGE_CURVE ( 'NONE', #3142, #1596, #1164, .T. ) ;
#17439=ADVANCED_FACE ( 'NONE', ( #7552 ), #1402, .T. ) ;
#17441=LINE ( 'NONE', #17157, #21220 ) ;
#17457=DIRECTION ( 'NONE',  ( 0.000000000000000000, 0.000000000000000000, 1.000000000000000000 ) ) ;
#17527=ORIENTED_EDGE ( 'NONE', *, *, #3170, .T. ) ;
#17544=VECTOR ( 'NONE', #20541, 1000.000000000000000 ) ;
#17551=CARTESIAN_POINT ( 'NONE',  ( 99.20899822134843760, 123.0000000000000000, -1.909647267044714436 ) ) ;
#17592=VERTEX_POINT ( 'NONE', #9232 ) ;
#17624=( BOUNDED_CURVE ( )  B_SPLINE_CURVE ( 2, ( #2368, #18424, #20424, #22849, #21896, #18283, #9722, #26989, #24697 ),
 .UNSPECIFIED., .F., .F. ) 
 B_SPLINE_CURVE_WITH_KNOTS ( ( 3, 2, 2, 2, 3 ),
 ( 0.5833333333333337034, 0.6250000000000002220, 0.6666666666666667407, 0.7083333333333332593, 0.7499999999999997780 ),
 .UNSPECIFIED. ) 
 CURVE ( )  GEOMETRIC_REPRESENTATION_ITEM ( )  RATIONAL_B_SPLINE_CURVE ( ( 0.9999999999999994449, 0.9238795325112872936, 1.000000000000000000, 0.9238795325112867385, 1.000000000000000000, 0.9238795325112867385, 1.000000000000000000, 0.9238795325112871826, 0.9999999999999995559 ) ) 
 REPRESENTATION_ITEM ( '' )  );
#17638=ADVANCED_FACE ( 'NONE', ( #4971 ), #12568, .T. ) ;
#17674=EDGE_CURVE ( 'NONE', #22175, #26480, #23330, .T. ) ;
#17699=CARTESIAN_POINT ( 'NONE',  ( 101.4615807364564546, 123.4500000010924765, 1.461580736456455476 ) ) ;
#17701=CARTESIAN_POINT ( 'NONE',  ( 99.37536711629694253, 123.0000000000000426, -2.000913270215707307 ) ) ;
#17725=CARTESIAN_POINT ( 'NONE',  ( 101.7677669529663547, 124.7000000000000028, -1.767766952966370209 ) ) ;
#17730=VECTOR ( 'NONE', #9711, 1000.000000000000000 ) ;
#17746=CARTESIAN_POINT ( 'NONE',  ( 97.50000000000000000, 125.0000000000000000, -9.540979117872439019E-15 ) ) ;
#17760=DIRECTION ( 'NONE',  ( 0.000000000000000000, 0.000000000000000000, 1.000000000000000000 ) ) ;
#17776=CIRCLE ( 'NONE', #19581, 11.50000000000001776 ) ;
#17805=EDGE_CURVE ( 'NONE', #9543, #15488, #18434, .T. ) ;
#17825=CARTESIAN_POINT ( 'NONE',  ( 102.0669872999999939, 124.3000000010924566, 0.8561741729129311862 ) ) ;
#17837=CARTESIAN_POINT ( 'NONE',  ( 97.93301270000000613, 124.7500000010924737, -9.540979117872439019E-15 ) ) ;
#17924=CARTESIAN_POINT ( 'NONE',  ( 101.4615807364564546, 123.2500000010924879, 1.461580736456455476 ) ) ;
#17943=ORIENTED_EDGE ( 'NONE', *, *, #23943, .F. ) ;
#17994=VECTOR ( 'NONE', #23519, 1000.000000000000000 ) ;
#18009=CARTESIAN_POINT ( 'NONE',  ( 99.99999999999998579, 124.7999999999999972, -2.499999999999997780 ) ) ;
#18019=EDGE_LOOP ( 'NONE', ( #12086, #21410 ) ) ;
#18062=CARTESIAN_POINT ( 'NONE',  ( 97.93301270000000613, 123.7500000010924879, -9.540979117872439019E-15 ) ) ;
#18093=CLOSED_SHELL ( 'NONE', ( #256, #3956, #11422, #17439, #27261, #4261, #12111, #2726, #23643, #1394, #4548, #16618, #23616, #2696, #12323, #2342, #4605, #19014, #6729, #8017, #12915, #17638, #5509, #16620 ) ) ;
#18144=ORIENTED_EDGE ( 'NONE', *, *, #3119, .F. ) ;
#18152=CARTESIAN_POINT ( 'NONE',  ( 97.93301270000000613, 122.9500000010924765, -9.540979117872439019E-15 ) ) ;
#18167=CARTESIAN_POINT ( 'NONE',  ( 100.8561741729129295, 123.5000000010924879, -2.066987299999998751 ) ) ;
#18176=STYLED_ITEM ( 'NONE', ( #20467 ), #24660 ) ;
#18212=CARTESIAN_POINT ( 'NONE',  ( 99.14382582708707048, 123.6000000010924680, -2.066987299999999195 ) ) ;
#18244=ORIENTED_EDGE ( 'NONE', *, *, #3119, .T. ) ;
#18283=CARTESIAN_POINT ( 'NONE',  ( 97.50000000000000000, 123.3499999999999943, -1.035533905932742416 ) ) ;
#18290=ORIENTED_EDGE ( 'NONE', *, *, #17674, .T. ) ;
#18298=CARTESIAN_POINT ( 'NONE',  ( 98.96446609406727646, 122.8500000021849416, 2.499999999999977796 ) ) ;
#18305=ORIENTED_EDGE ( 'NONE', *, *, #17805, .T. ) ;
#18317=DIRECTION ( 'NONE',  ( 0.000000000000000000, 1.000000000000000000, 0.000000000000000000 ) ) ;
#18362=EDGE_CURVE ( 'NONE', #13578, #9543, #23913, .T. ) ;
#18398=CARTESIAN_POINT ( 'NONE',  ( 99.99999999999998579, 124.0000000000000000, -2.499999999999997780 ) ) ;
#18403=CARTESIAN_POINT ( 'NONE',  ( 99.99999999999998579, 138.0000000000000000, -5.204170427930421283E-15 ) ) ;
#18407=PLANE ( 'NONE',  #24388 ) ;
#18424=CARTESIAN_POINT ( 'NONE',  ( 98.96446609406726225, 123.5500000000000114, 2.499999999999972022 ) ) ;
#18434=( BOUNDED_CURVE ( )  B_SPLINE_CURVE ( 2, ( #26159, #11170, #21609, #24169, #4646, #8634, #6627, #26452, #12748 ),
 .UNSPECIFIED., .F., .F. ) 
 B_SPLINE_CURVE_WITH_KNOTS ( ( 3, 2, 2, 2, 3 ),
 ( 0.2499999999999998335, 0.2916666666666665741, 0.3333333333333332593, 0.3750000000000000000, 0.4166666666666667407 ),
 .UNSPECIFIED. ) 
 CURVE ( )  GEOMETRIC_REPRESENTATION_ITEM ( )  RATIONAL_B_SPLINE_CURVE ( ( 1.000000000000000222, 0.9238795325112864054, 1.000000000000000000, 0.9238795325112867385, 1.000000000000000000, 0.9238795325112867385, 1.000000000000000000, 0.9238795325112866275, 1.000000000000000000 ) ) 
 REPRESENTATION_ITEM ( '' )  );
#18445=CARTESIAN_POINT ( 'NONE',  ( 101.0355339059327378, 123.2500000021849758, -2.499999999999997780 ) ) ;
#18459=CARTESIAN_POINT ( 'NONE',  ( 99.14382582708708469, 123.6000000010924680, -2.066987299999998751 ) ) ;
#18489=ORIENTED_EDGE ( 'NONE', *, *, #27805, .T. ) ;
#18514=EDGE_LOOP ( 'NONE', ( #6685, #13328, #14508, #10254 ) ) ;
#18541=CARTESIAN_POINT ( 'NONE',  ( 100.8561741729129295, 123.4000000010924794, 2.066987299999979211 ) ) ;
#18549=FACE_BOUND ( 'NONE', #4890, .T. ) ;
#18579=CARTESIAN_POINT ( 'NONE',  ( 99.99999999999998579, 138.0000000000000000, -11.50000000000002309 ) ) ;
#18580=VERTEX_POINT ( 'NONE', #28109 ) ;
#18582=CARTESIAN_POINT ( 'NONE',  ( 97.50000000000000000, 122.6500000021849530, -1.035533905932742416 ) ) ;
#18638=CARTESIAN_POINT ( 'NONE',  ( 102.0669872999999797, 124.3500000010924822, -9.794112055954760458E-15 ) ) ;
#18649=LINE ( 'NONE', #7812, #17206 ) ;
#18680=CARTESIAN_POINT ( 'NONE',  ( 97.93301269999999192, 124.0000000010924879, 0.8561741729129329626 ) ) ;
#18715=AXIS2_PLACEMENT_3D ( 'NONE', #27426, #16584, #25277 ) ;
#18720=CARTESIAN_POINT ( 'NONE',  ( 99.99999999999998579, 123.9500000010924765, 2.066987299999980099 ) ) ;
#18722=CARTESIAN_POINT ( 'NONE',  ( 98.09035273295538104, 123.0000000000000142, 0.7910017786517971050 ) ) ;
#18728=CYLINDRICAL_SURFACE ( 'NONE', #18715, 12.50000000000001599 ) ;
#18747=CARTESIAN_POINT ( 'NONE',  ( 99.99999999999998579, 128.0000000000000000, -5.204170427930421283E-15 ) ) ;
#18765=LINE ( 'NONE', #18894, #13406 ) ;
#18772=CARTESIAN_POINT ( 'NONE',  ( 99.14382582708707048, 124.6000000010924822, -2.066987299999999195 ) ) ;
#18811=CARTESIAN_POINT ( 'NONE',  ( 97.93301269999999192, 123.9000000010924794, -0.8561741729129505041 ) ) ;
#18831=ORIENTED_EDGE ( 'NONE', *, *, #18939, .F. ) ;
#18854=CARTESIAN_POINT ( 'NONE',  ( 102.4999999999999858, 123.0000000000000000, -8.724596124144689908E-15 ) ) ;
#18860=VERTEX_POINT ( 'NONE', #24681 ) ;
#18871=( NAMED_UNIT ( * ) PLANE_ANGLE_UNIT ( ) SI_UNIT ( $, .RADIAN. ) );
#18872=CARTESIAN_POINT ( 'NONE',  ( 99.99999999999998579, 123.0000000000000000, -5.204170427930421283E-15 ) ) ;
#18894=CARTESIAN_POINT ( 'NONE',  ( 99.99999999999998579, 128.0000000000000000, 2.500000000000003553 ) ) ;
#18903=CARTESIAN_POINT ( 'NONE',  ( 101.4615807364564546, 124.4500000010924765, -1.461580736456474794 ) ) ;
#18907=CYLINDRICAL_SURFACE ( 'NONE', #774, 2.500000000000008882 ) ;
#18915=DIRECTION ( 'NONE',  ( 0.8660254037844380415, 0.5000000000000013323, 0.000000000000000000 ) ) ;
#18939=EDGE_CURVE ( 'NONE', #17592, #8172, #11971, .T. ) ;
#18945=CARTESIAN_POINT ( 'NONE',  ( 99.14382582708707048, 123.8000000010924850, -2.066987299999999195 ) ) ;
#18997=DIRECTION ( 'NONE',  ( 0.000000000000000000, -0.000000000000000000, 1.000000000000000000 ) ) ;
#19014=ADVANCED_FACE ( 'NONE', ( #18549, #3582 ), #18407, .T. ) ;
#19028=CARTESIAN_POINT ( 'NONE',  ( 99.99999999999998579, 136.0000000000000000, -5.204170427930421283E-15 ) ) ;
#19135=CARTESIAN_POINT ( 'NONE',  ( 100.0265503228089301, 123.0000000000000426, 2.336440708561638768 ) ) ;
#19144=EDGE_LOOP ( 'NONE', ( #329, #24370, #603, #825 ) ) ;
#19184=CARTESIAN_POINT ( 'NONE',  ( 98.53841926354351699, 123.0500000010924850, -1.461580736456474794 ) ) ;
#19186=ORIENTED_EDGE ( 'NONE', *, *, #7742, .F. ) ;
#19225=CARTESIAN_POINT ( 'NONE',  ( 97.93301270000000613, 124.5500000010924850, -9.540979117872439019E-15 ) ) ;
#19265=VECTOR ( 'NONE', #22808, 1000.000000000000000 ) ;
#19274=EDGE_CURVE ( 'NONE', #6030, #24651, #25382, .T. ) ;
#19412=CARTESIAN_POINT ( 'NONE',  ( 99.84091028936038015, 123.0000000000000000, 2.314727449556549299 ) ) ;
#19448=EDGE_CURVE ( 'NONE', #15488, #2621, #13786, .T. ) ;
#19554=CARTESIAN_POINT ( 'NONE',  ( 100.8561741729129437, 123.4000000010924509, 2.066987299999979655 ) ) ;
#19581=AXIS2_PLACEMENT_3D ( 'NONE', #20399, #884, #4871 ) ;
#19598=EDGE_CURVE ( 'NONE', #6493, #10914, #27575, .T. ) ;
#19621=LINE ( 'NONE', #9211, #15125 ) ;
#19653=CARTESIAN_POINT ( 'NONE',  ( 98.03825896092904202, 123.0000000000000142, -0.6650219646036082954 ) ) ;
#19676=ORIENTED_EDGE ( 'NONE', *, *, #14713, .F. ) ;
#19691=CARTESIAN_POINT ( 'NONE',  ( 100.8561741729129295, 123.7000000010924765, -2.066987299999998751 ) ) ;
#19836=CARTESIAN_POINT ( 'NONE',  ( 99.99999999999998579, 136.0000000000000000, -10.50000000000002132 ) ) ;
#19881=AXIS2_PLACEMENT_3D ( 'NONE', #14142, #11716, #5049 ) ;
#19985=CARTESIAN_POINT ( 'NONE',  ( 99.14382582708708469, 124.6000000010924822, -2.066987299999998751 ) ) ;
#20016=( GEOMETRIC_REPRESENTATION_CONTEXT ( 3 ) GLOBAL_UNCERTAINTY_ASSIGNED_CONTEXT ( ( #8982 ) ) GLOBAL_UNIT_ASSIGNED_CONTEXT ( ( #9848, #24538, #22839 ) ) REPRESENTATION_CONTEXT ( 'NONE', 'WORKASPACE' ) );
#20052=DIRECTION ( 'NONE',  ( 0.000000000000000000, 0.000000000000000000, 1.000000000000000000 ) ) ;
#20088=CARTESIAN_POINT ( 'NONE',  ( 98.44193425395140196, 123.0000000000000711, -1.364916718493922820 ) ) ;
#20093=AXIS2_PLACEMENT_3D ( 'NONE', #10722, #23850, #15420 ) ;
#20131=EDGE_CURVE ( 'NONE', #13199, #20976, #7636, .T. ) ;
#20168=ORIENTED_EDGE ( 'NONE', *, *, #12792, .F. ) ;
#20205=CARTESIAN_POINT ( 'NONE',  ( 102.4999999999999858, 123.0000000000000000, -8.724596124144689908E-15 ) ) ;
#20295=CARTESIAN_POINT ( 'NONE',  ( 100.8561741729129153, 123.5000000010924737, -2.066987299999999195 ) ) ;
#20309=CARTESIAN_POINT ( 'NONE',  ( 99.14382582708708469, 123.9000000010924794, 2.066987299999979655 ) ) ;
#20358=CARTESIAN_POINT ( 'NONE',  ( 101.7677669529663547, 123.2000000021849502, -1.767766952966370209 ) ) ;
#20399=CARTESIAN_POINT ( 'NONE',  ( 99.99999999999998579, 138.0000000000000000, -5.204170427930421283E-15 ) ) ;
#20411=SURFACE_STYLE_USAGE ( .BOTH. , #11687 ) ;
#20424=CARTESIAN_POINT ( 'NONE',  ( 98.23223304703363112, 123.5000000000000000, 1.767766952966351557 ) ) ;
#20444=CARTESIAN_POINT ( 'NONE',  ( 101.4615807364564546, 124.0500000010924850, 1.461580736456455476 ) ) ;
#20467=PRESENTATION_STYLE_ASSIGNMENT (( #7476 ) ) ;
#20482=CARTESIAN_POINT ( 'NONE',  ( 99.99999999999998579, 129.0000000000000000, -5.204170427930421283E-15 ) ) ;
#20493=EDGE_CURVE ( 'NONE', #13180, #2621, #17441, .T. ) ;
#20541=DIRECTION ( 'NONE',  ( -0.000000000000000000, -1.000000000000000000, -0.000000000000000000 ) ) ;
#20545=CARTESIAN_POINT ( 'NONE',  ( 98.23223304703363112, 124.2999999999999972, 1.767766952966351557 ) ) ;
#20557=VERTEX_POINT ( 'NONE', #10598 ) ;
#20585=CARTESIAN_POINT ( 'NONE',  ( 102.4999999999999858, 122.3000000021849587, -9.847140817659276890E-15 ) ) ;
#20630=ORIENTED_EDGE ( 'NONE', *, *, #16138, .T. ) ;
#20640=CARTESIAN_POINT ( 'NONE',  ( 102.0669872999999939, 124.1000000010924964, 0.8561741729129311862 ) ) ;
#20663=EDGE_CURVE ( 'NONE', #487, #13578, #9808, .T. ) ;
#20679=DIRECTION ( 'NONE',  ( -0.000000000000000000, 1.000000000000000000, -0.000000000000000000 ) ) ;
#20685=CARTESIAN_POINT ( 'NONE',  ( 99.99999999999998579, 123.6000000000000085, 2.499999999999978684 ) ) ;
#20726=CARTESIAN_POINT ( 'NONE',  ( 101.7677669529663547, 123.0000000021849615, 1.767766952966350891 ) ) ;
#20821=CARTESIAN_POINT ( 'NONE',  ( 101.4615807364564546, 123.6500000010924651, -1.461580736456474794 ) ) ;
#20853=EDGE_CURVE ( 'NONE', #10914, #20981, #17161, .T. ) ;
#20863=CARTESIAN_POINT ( 'NONE',  ( 99.99999999999998579, 122.9000000021849530, 2.499999999999978684 ) ) ;
#20881=DIRECTION ( 'NONE',  ( 0.000000000000000000, 1.000000000000000000, 0.000000000000000000 ) ) ;
#20892=PLANE ( 'NONE',  #27647 ) ;
#20918=CARTESIAN_POINT ( 'NONE',  ( 99.99999999999998579, 124.1500000010924651, 2.066987299999980099 ) ) ;
#20936=EDGE_LOOP ( 'NONE', ( #25601, #1562, #14234, #4104 ) ) ;
#20958=CARTESIAN_POINT ( 'NONE',  ( 101.0355339059327378, 124.4500000000000028, 2.499999999999977796 ) ) ;
#20968=DIRECTION ( 'NONE',  ( 0.000000000000000000, 1.000000000000000000, 0.000000000000000000 ) ) ;
#20976=VERTEX_POINT ( 'NONE', #15801 ) ;
#20978=EDGE_LOOP ( 'NONE', ( #13553, #6354, #23575, #565 ) ) ;
#20981=VERTEX_POINT ( 'NONE', #12836 ) ;
#20998=CARTESIAN_POINT ( 'NONE',  ( 99.99999999999998579, 128.0000000000000000, -5.204170427930421283E-15 ) ) ;
#21048=CARTESIAN_POINT ( 'NONE',  ( 97.50000000000000000, 123.5500000021849587, 1.035533905932725096 ) ) ;
#21050=LINE ( 'NONE', #25879, #7621 ) ;
#21055=CARTESIAN_POINT ( 'NONE',  ( 98.53841926354351699, 124.6500000010924651, -1.461580736456474794 ) ) ;
#21082=AXIS2_PLACEMENT_3D ( 'NONE', #4806, #2391, #20052 ) ;
#21093=CARTESIAN_POINT ( 'NONE',  ( 102.4999999999999858, 124.6000000000000085, -9.847140817659276890E-15 ) ) ;
#21125=CARTESIAN_POINT ( 'NONE',  ( 101.7677669529663547, 123.0999999999999943, -1.767766952966370209 ) ) ;
#21135=ORIENTED_EDGE ( 'NONE', *, *, #25892, .T. ) ;
#21197=CARTESIAN_POINT ( 'NONE',  ( 99.20899822134843760, 123.0000000000000000, -1.909647267044714436 ) ) ;
#21220=VECTOR ( 'NONE', #2210, 1000.000000000000000 ) ;
#21229=CARTESIAN_POINT ( 'NONE',  ( 99.99999999999998579, 138.0000000000000000, -5.204170427930421283E-15 ) ) ;
#21248=CARTESIAN_POINT ( 'NONE',  ( 98.96446609406724804, 124.1500000021849672, -2.499999999999992450 ) ) ;
#21333=CARTESIAN_POINT ( 'NONE',  ( 97.93301269999999192, 124.7000000010924623, -0.8561741729129505041 ) ) ;
#21365=EDGE_CURVE ( 'NONE', #14731, #25689, #4391, .T. ) ;
#21397=EDGE_LOOP ( 'NONE', ( #26565, #16859, #18290, #10362 ) ) ;
#21410=ORIENTED_EDGE ( 'NONE', *, *, #27520, .F. ) ;
#21484=CARTESIAN_POINT ( 'NONE',  ( 101.9991671059954683, 123.0000000000000142, 1.536366799937288974 ) ) ;
#21547=AXIS2_PLACEMENT_3D ( 'NONE', #23568, #12564, #7895 ) ;
#21609=CARTESIAN_POINT ( 'NONE',  ( 98.23223304703363112, 124.2999999999999972, 1.767766952966351557 ) ) ;
#21610=AXIS2_PLACEMENT_3D ( 'NONE', #12563, #23014, #3345 ) ;
#21631=LINE ( 'NONE', #4383, #6289 ) ;
#21661=CARTESIAN_POINT ( 'NONE',  ( 101.7677669529663547, 123.8999999999999915, -1.767766952966370209 ) ) ;
#21702=CARTESIAN_POINT ( 'NONE',  ( 100.8561741729129437, 124.2000000010924623, 2.066987299999979655 ) ) ;
#21724=CYLINDRICAL_SURFACE ( 'NONE', #20093, 2.500000000000008882 ) ;
#21796=CARTESIAN_POINT ( 'NONE',  ( 99.99999999999998579, 123.2000000000000028, -2.499999999999997780 ) ) ;
#21805=CARTESIAN_POINT ( 'NONE',  ( 99.99999999999998579, 124.0000000000000000, -2.499999999999997780 ) ) ;
#21853=CARTESIAN_POINT ( 'NONE',  ( 97.71650635000000307, 124.8750000005462368, -9.540979117872439019E-15 ) ) ;
#21874=EDGE_CURVE ( 'NONE', #6277, #8833, #6217, .T. ) ;
#21896=CARTESIAN_POINT ( 'NONE',  ( 97.50000000000000000, 123.3999999999999915, -9.540979117872439019E-15 ) ) ;
#22085=CARTESIAN_POINT ( 'NONE',  ( 98.20479815727543382, 122.9999999999999432, -1.033452060272729067 ) ) ;
#22112=CARTESIAN_POINT ( 'NONE',  ( 101.4615807364564546, 124.4500000010924765, -1.461580736456474794 ) ) ;
#22158=ORIENTED_EDGE ( 'NONE', *, *, #20853, .T. ) ;
#22166=CARTESIAN_POINT ( 'NONE',  ( 101.4615807364564546, 124.2500000010924879, -1.461580736456474794 ) ) ;
#22168=CARTESIAN_POINT ( 'NONE',  ( 101.0355339059327235, 123.7500000021849615, 2.499999999999987121 ) ) ;
#22175=VERTEX_POINT ( 'NONE', #22707 ) ;
#22212=CARTESIAN_POINT ( 'NONE',  ( 101.0355339059327235, 123.2500000021849615, -2.499999999999998668 ) ) ;
#22227=CARTESIAN_POINT ( 'NONE',  ( 99.99999999999998579, 123.6000000000000085, 2.499999999999978684 ) ) ;
#22272=EDGE_CURVE ( 'NONE', #2621, #20557, #17624, .T. ) ;
#22322=ORIENTED_EDGE ( 'NONE', *, *, #23440, .T. ) ;
#22331=VECTOR ( 'NONE', #12464, 999.9999999999998863 ) ;
#22365=ORIENTED_EDGE ( 'NONE', *, *, #12527, .T. ) ;
#22379=DIRECTION ( 'NONE',  ( 0.000000000000000000, 0.000000000000000000, 1.000000000000000000 ) ) ;
#22393=FACE_OUTER_BOUND ( 'NONE', #23946, .T. ) ;
#22439=CARTESIAN_POINT ( 'NONE',  ( 102.0669872999999797, 123.3500000010924680, -9.794112055954760458E-15 ) ) ;
#22451=CARTESIAN_POINT ( 'NONE',  ( 98.53841926354351699, 123.0500000010924850, 1.461580736456455920 ) ) ;
#22453=APPLICATION_CONTEXT ( 'automotive_design' ) ;
#22474=DIRECTION ( 'NONE',  ( -0.000000000000000000, -1.000000000000000000, -0.000000000000000000 ) ) ;
#22490=DIRECTION ( 'NONE',  ( 8.659560562354941486E-17, 0.7071067811865469066, -0.7071067811865482389 ) ) ;
#22492=DIRECTION ( 'NONE',  ( 0.000000000000000000, 0.000000000000000000, -1.000000000000000000 ) ) ;
#22493=CARTESIAN_POINT ( 'NONE',  ( 101.4615807364564546, 124.2500000010924879, -1.461580736456474794 ) ) ;
#22515=EDGE_CURVE ( 'NONE', #20976, #26480, #10148, .T. ) ;
#22549=DIRECTION ( 'NONE',  ( 0.000000000000000000, 0.000000000000000000, -1.000000000000000000 ) ) ;
#22559=ORIENTED_EDGE ( 'NONE', *, *, #9787, .T. ) ;
#22578=CYLINDRICAL_SURFACE ( 'NONE', #19881, 2.500000000000008882 ) ;
#22582=CARTESIAN_POINT ( 'NONE',  ( 98.53841926354351699, 122.8500000010924680, -1.461580736456474794 ) ) ;
#22606=ORIENTED_EDGE ( 'NONE', *, *, #19274, .T. ) ;
#22641=CARTESIAN_POINT ( 'NONE',  ( 100.8561741729129295, 123.2000000010924765, 2.066987299999979211 ) ) ;
#22683=CARTESIAN_POINT ( 'NONE',  ( 97.93301270000000613, 123.1500000010924651, -9.540979117872439019E-15 ) ) ;
#22707=CARTESIAN_POINT ( 'NONE',  ( 99.99999999999998579, 128.0000000000000000, 11.50000000000000888 ) ) ;
#22725=CARTESIAN_POINT ( 'NONE',  ( 99.99999999999998579, 122.5000000021849615, -2.499999999999997780 ) ) ;
#22748=( NAMED_UNIT ( * ) SI_UNIT ( $, .STERADIAN. ) SOLID_ANGLE_UNIT ( ) );
#22749=( GEOMETRIC_REPRESENTATION_CONTEXT ( 3 ) GLOBAL_UNCERTAINTY_ASSIGNED_CONTEXT ( ( #12586 ) ) GLOBAL_UNIT_ASSIGNED_CONTEXT ( ( #16738, #9618, #3215 ) ) REPRESENTATION_CONTEXT ( 'NONE', 'WORKASPACE' ) );
#22782=CARTESIAN_POINT ( 'NONE',  ( 98.53841926354351699, 123.8500000010924680, 1.461580736456455920 ) ) ;
#22808=DIRECTION ( 'NONE',  ( -0.000000000000000000, -1.000000000000000000, -0.000000000000000000 ) ) ;
#22825=CARTESIAN_POINT ( 'NONE',  ( 98.53841926354351699, 123.8500000010924680, -1.461580736456474794 ) ) ;
#22839=( NAMED_UNIT ( * ) SI_UNIT ( $, .STERADIAN. ) SOLID_ANGLE_UNIT ( ) );
#22849=CARTESIAN_POINT ( 'NONE',  ( 97.50000000000000000, 123.4500000000000028, 1.035533905932725096 ) ) ;
#22864=CARTESIAN_POINT ( 'NONE',  ( 97.93301269999999192, 122.9000000010924936, -0.8561741729129505041 ) ) ;
#22873=FACE_OUTER_BOUND ( 'NONE', #7592, .T. ) ;
#22879=CARTESIAN_POINT ( 'NONE',  ( 99.99999999999998579, 123.0000000000000000, 0.5000000000000034417 ) ) ;
#22886=ORIENTED_EDGE ( 'NONE', *, *, #324, .F. ) ;
#22915=ORIENTED_EDGE ( 'NONE', *, *, #26645, .F. ) ;
#22922=CARTESIAN_POINT ( 'NONE',  ( 102.0669872999999939, 122.6000000010924964, -0.8561741729129507261 ) ) ;
#22965=CARTESIAN_POINT ( 'NONE',  ( 99.14382582708707048, 123.3000000010924708, 2.066987299999979211 ) ) ;
#23001=CARTESIAN_POINT ( 'NONE',  ( 98.23223304703363112, 123.4000000021849530, -1.767766952966370209 ) ) ;
#23004=LINE ( 'NONE', #3474, #15786 ) ;
#23010=CARTESIAN_POINT ( 'NONE',  ( 97.50000000000000000, 124.3000000021849587, -9.540979117872439019E-15 ) ) ;
#23014=DIRECTION ( 'NONE',  ( -0.000000000000000000, -1.000000000000000000, -0.000000000000000000 ) ) ;
#23046=FACE_OUTER_BOUND ( 'NONE', #10702, .T. ) ;
#23049=FACE_OUTER_BOUND ( 'NONE', #11843, .T. ) ;
#23055=CARTESIAN_POINT ( 'NONE',  ( 102.0669872999999939, 122.8000000010924708, -0.8561741729129507261 ) ) ;
#23091=AXIS2_PLACEMENT_3D ( 'NONE', #23978, #17270, #4455 ) ;
#23098=CARTESIAN_POINT ( 'NONE',  ( 102.4999999999999716, 123.7500000000000142, 1.035533905932722876 ) ) ;
#23148=VERTEX_POINT ( 'NONE', #20205 ) ;
#23151=CIRCLE ( 'NONE', #12663, 11.50000000000001421 ) ;
#23158=CARTESIAN_POINT ( 'NONE',  ( 99.99999999999998579, 124.1000000021849416, -2.499999999999997780 ) ) ;
#23163=FILL_AREA_STYLE ('',( #27582 ) ) ;
#23186=DIRECTION ( 'NONE',  ( 0.000000000000000000, -0.000000000000000000, 1.000000000000000000 ) ) ;
#23189=CARTESIAN_POINT ( 'NONE',  ( 99.99999999999998579, 123.7000000021849502, 2.499999999999978684 ) ) ;
#23193=COLOUR_RGB ( '', 0.31764706, 0.68627451, 0.89019608) ;
#23198=CARTESIAN_POINT ( 'NONE',  ( 102.0669872999999939, 123.5000000010924595, 0.8561741729129311862 ) ) ;
#23207=CARTESIAN_POINT ( 'NONE',  ( 97.71650635000000307, 124.4250000016387219, -9.540979117872439019E-15 ) ) ;
#23236=CARTESIAN_POINT ( 'NONE',  ( 97.93301269999999192, 123.1000000010924822, -0.8561741729129505041 ) ) ;
#23300=CARTESIAN_POINT ( 'NONE',  ( 99.99999999999998579, 130.0000000000000000, -5.204170427930421283E-15 ) ) ;
#23305=SURFACE_SIDE_STYLE ('',( #3639 ) ) ;
#23330=LINE ( 'NONE', #8348, #22331 ) ;
#23386=AXIS2_PLACEMENT_3D ( 'NONE', #16802, #20679, #7834 ) ;
#23389=DIRECTION ( 'NONE',  ( -0.000000000000000000, -1.000000000000000000, -0.000000000000000000 ) ) ;
#23420=CARTESIAN_POINT ( 'NONE',  ( 101.0282581911821040, 123.0000000000000142, -2.018985708853541894 ) ) ;
#23440=EDGE_CURVE ( 'NONE', #1596, #18580, #23842, .T. ) ;
#23489=CARTESIAN_POINT ( 'NONE',  ( 99.99999999999998579, 123.0000000000000000, -0.5000000000000138778 ) ) ;
#23505=DIRECTION ( 'NONE',  ( -0.000000000000000000, -1.000000000000000000, -0.000000000000000000 ) ) ;
#23519=DIRECTION ( 'NONE',  ( 0.000000000000000000, 1.000000000000000000, 0.000000000000000000 ) ) ;
#23525=ORIENTED_EDGE ( 'NONE', *, *, #25892, .F. ) ;
#23568=CARTESIAN_POINT ( 'NONE',  ( 99.99999999999998579, 136.0000000000000000, -5.204170427930421283E-15 ) ) ;
#23575=ORIENTED_EDGE ( 'NONE', *, *, #10051, .T. ) ;
#23608=DIRECTION ( 'NONE',  ( 1.000000000000000000, 0.000000000000000000, 0.000000000000000000 ) ) ;
#23616=ADVANCED_FACE ( 'NONE', ( #24167 ), #513, .T. ) ;
#23623=( BOUNDED_CURVE ( )  B_SPLINE_CURVE ( 2, ( #17837, #4736, #319, #19985, #6856, #13107, #463, #24114, #35, #6442, #178, #21702, #10979, #8578, #2322, #4882, #17268, #10840, #9144, #2035, #25969, #19691, #8860, #23832, #28114, #26542, #17699, #19554, #6998, #15257, #4591, #13546, #24394, #15546, #24254, #12970, #17551 ),
 .UNSPECIFIED., .F., .F. ) 
 B_SPLINE_CURVE_WITH_KNOTS ( ( 3, 2, 2, 2, 2, 2, 2, 2, 2, 2, 2, 2, 2, 2, 2, 2, 2, 2, 3 ),
 ( 0.000000000000000000, 0.04166666666666666435, 0.08333333333333332871, 0.1250000000000000000, 0.1666666666666666574, 0.2083333333333333148, 0.2500000000000000000, 0.2916666666666666852, 0.3333333333333333148, 0.3750000000000000000, 0.4166666666666666297, 0.4583333333333333148, 0.5000000000000000000, 0.5416666666666666297, 0.5833333333333333703, 0.6250000000000000000, 0.6666666666666666297, 0.7083333333333334814, 0.7291666671045423653 ),
 .UNSPECIFIED. ) 
 CURVE ( )  GEOMETRIC_REPRESENTATION_ITEM ( )  RATIONAL_B_SPLINE_CURVE ( ( 1.000000000000000000, 0.9238795325112867385, 1.000000000000000000, 0.9238795325112867385, 1.000000000000000000, 0.9238795325112867385, 1.000000000000000000, 0.9238795325112867385, 1.000000000000000000, 0.9238795325112867385, 1.000000000000000000, 0.9238795325112867385, 1.000000000000000000, 0.9238795325112867385, 1.000000000000000000, 0.9238795325112867385, 1.000000000000000000, 0.9238795325112867385, 1.000000000000000000, 0.9238795325112867385, 1.000000000000000000, 0.9238795325112867385, 1.000000000000000000, 0.9238795325112867385, 1.000000000000000000, 0.9238795325112867385, 1.000000000000000000, 0.9238795325112867385, 1.000000000000000000, 0.9238795325112867385, 1.000000000000000000, 0.9238795325112867385, 1.000000000000000000, 0.9238795325112867385, 1.000000000000000000, 0.9619397654556921529, 0.9619397662556433692 ) ) 
 REPRESENTATION_ITEM ( '' )  );
#23643=ADVANCED_FACE ( 'NONE', ( #13445 ), #224, .T. ) ;
#23713=AXIS2_PLACEMENT_3D ( 'NONE', #21853, #18997, #1768 ) ;
#23720=DIRECTION ( 'NONE',  ( 0.000000000000000000, 1.000000000000000000, 0.000000000000000000 ) ) ;
#23744=CARTESIAN_POINT ( 'NONE',  ( 99.99999999999998579, 130.0000000000000000, -5.204170427930421283E-15 ) ) ;
#23757=CARTESIAN_POINT ( 'NONE',  ( 99.99999999999998579, 124.7999999999999972, -2.499999999999997780 ) ) ;
#23821=CIRCLE ( 'NONE', #21547, 10.50000000000001599 ) ;
#23831=VERTEX_POINT ( 'NONE', #23158 ) ;
#23832=CARTESIAN_POINT ( 'NONE',  ( 102.0669873000000081, 123.6000000010924680, -0.8561741729129508371 ) ) ;
#23834=CARTESIAN_POINT ( 'NONE',  ( 99.47614712164786965, 123.0000000000000000, 2.223611564848176236 ) ) ;
#23842=CIRCLE ( 'NONE', #7437, 10.50000000000001599 ) ;
#23850=DIRECTION ( 'NONE',  ( -0.000000000000000000, -1.000000000000000000, -0.000000000000000000 ) ) ;
#23913=( BOUNDED_CURVE ( )  B_SPLINE_CURVE ( 2, ( #28138, #13276, #17725, #4335, #6325, #12855, #24140, #2348, #4196 ),
 .UNSPECIFIED., .F., .F. ) 
 B_SPLINE_CURVE_WITH_KNOTS ( ( 3, 2, 2, 2, 3 ),
 ( 0.08333333333333389770, 0.1250000000000003886, 0.1666666666666668517, 0.2083333333333333426, 0.2499999999999998335 ),
 .UNSPECIFIED. ) 
 CURVE ( )  GEOMETRIC_REPRESENTATION_ITEM ( )  RATIONAL_B_SPLINE_CURVE ( ( 0.9999999999999990008, 0.9238795325112877377, 1.000000000000000000, 0.9238795325112867385, 1.000000000000000000, 0.9238795325112867385, 1.000000000000000000, 0.9238795325112870716, 0.9999999999999996669 ) ) 
 REPRESENTATION_ITEM ( '' )  );
#23920=EDGE_CURVE ( 'NONE', #8833, #6277, #11018, .T. ) ;
#23943=EDGE_CURVE ( 'NONE', #1875, #17592, #8309, .T. ) ;
#23946=EDGE_LOOP ( 'NONE', ( #18244, #19186, #18489, #15315, #3344, #18305, #24962, #2286, #1546 ) ) ;
#23978=CARTESIAN_POINT ( 'NONE',  ( 99.99999999999998579, 137.0000000000000000, -5.204170427930421283E-15 ) ) ;
#23998=EDGE_LOOP ( 'NONE', ( #26726, #24173, #3163, #26741 ) ) ;
#24028=DIRECTION ( 'NONE',  ( 0.000000000000000000, 0.000000000000000000, 1.000000000000000000 ) ) ;
#24114=CARTESIAN_POINT ( 'NONE',  ( 102.0669873000000081, 124.4000000010924651, -0.8561741729129508371 ) ) ;
#24140=CARTESIAN_POINT ( 'NONE',  ( 101.7677669529663547, 124.5000000000000000, 1.767766952966350891 ) ) ;
#24167=FACE_OUTER_BOUND ( 'NONE', #8494, .T. ) ;
#24169=CARTESIAN_POINT ( 'NONE',  ( 97.50000000000000000, 124.2500000000000000, 1.035533905932725096 ) ) ;
#24173=ORIENTED_EDGE ( 'NONE', *, *, #15657, .T. ) ;
#24218=CARTESIAN_POINT ( 'NONE',  ( 101.0355339059327235, 123.9500000000000028, -2.499999999999996447 ) ) ;
#24228=ORIENTED_EDGE ( 'NONE', *, *, #15195, .F. ) ;
#24254=CARTESIAN_POINT ( 'NONE',  ( 98.53841926354351699, 123.0500000010924850, -1.461580736456474794 ) ) ;
#24302=DIRECTION ( 'NONE',  ( 0.000000000000000000, -0.000000000000000000, 1.000000000000000000 ) ) ;
#24336=AXIS2_PLACEMENT_3D ( 'NONE', #3662, #1252, #14468 ) ;
#24353=ORIENTED_EDGE ( 'NONE', *, *, #19598, .F. ) ;
#24368=CARTESIAN_POINT ( 'NONE',  ( 99.99999999999998579, 138.0000000000000000, 11.50000000000001243 ) ) ;
#24370=ORIENTED_EDGE ( 'NONE', *, *, #15750, .T. ) ;
#24388=AXIS2_PLACEMENT_3D ( 'NONE', #1590, #20968, #3437 ) ;
#24394=CARTESIAN_POINT ( 'NONE',  ( 97.93301270000000613, 123.1500000010924651, -9.540979117872439019E-15 ) ) ;
#24432=ORIENTED_EDGE ( 'NONE', *, *, #20493, .T. ) ;
#24438=CARTESIAN_POINT ( 'NONE',  ( 101.4615807364564546, 123.4500000010924765, -1.461580736456474794 ) ) ;
#24440=CARTESIAN_POINT ( 'NONE',  ( 101.7677669529663547, 124.0000000021849615, -1.767766952966370209 ) ) ;
#24505=CARTESIAN_POINT ( 'NONE',  ( 101.6232090348605510, 123.0000000000000426, 1.890011928979586697 ) ) ;
#24509=EDGE_CURVE ( 'NONE', #11544, #20981, #2577, .T. ) ;
#24538=( NAMED_UNIT ( * ) PLANE_ANGLE_UNIT ( ) SI_UNIT ( $, .RADIAN. ) );
#24572=MECHANICAL_DESIGN_GEOMETRIC_PRESENTATION_REPRESENTATION('',(#11342),#20016);
#24651=VERTEX_POINT ( 'NONE', #11495 ) ;
#24660=ADVANCED_BREP_SHAPE_REPRESENTATION ( '', ( #7835, #26844 ), #7245 ) ;
#24663=ORIENTED_EDGE ( 'NONE', *, *, #23920, .T. ) ;
#24673=CARTESIAN_POINT ( 'NONE',  ( 99.99999999999998579, 124.5500000010924708, -2.066987299999998751 ) ) ;
#24681=CARTESIAN_POINT ( 'NONE',  ( 99.99999999999998579, 128.0000000000000000, -11.50000000000001954 ) ) ;
#24697=CARTESIAN_POINT ( 'NONE',  ( 99.99999999999998579, 123.2000000000000028, -2.499999999999997780 ) ) ;
#24715=CARTESIAN_POINT ( 'NONE',  ( 99.99999999999998579, 124.3500000010924822, -2.066987299999998751 ) ) ;
#24768=CARTESIAN_POINT ( 'NONE',  ( 100.8561741729129153, 123.5000000010924737, -2.066987299999999195 ) ) ;
#24809=CARTESIAN_POINT ( 'NONE',  ( 99.99999999999998579, 123.7500000010924737, -2.066987299999998751 ) ) ;
#24821=CARTESIAN_POINT ( 'NONE',  ( 99.99999999999998579, 138.0000000000000000, 10.50000000000001066 ) ) ;
#24855=CARTESIAN_POINT ( 'NONE',  ( 102.4999999999999716, 123.1500000021849672, -1.035533905932742638 ) ) ;
#24856=CARTESIAN_POINT ( 'NONE',  ( 97.50000000000000000, 125.0000000000000000, -9.540979117872439019E-15 ) ) ;
#24868=CARTESIAN_POINT ( 'NONE',  ( 102.0669872999999797, 124.1500000010924794, -9.794112055954760458E-15 ) ) ;
#24881=EDGE_LOOP ( 'NONE', ( #22559, #3509 ) ) ;
#24892=DIRECTION ( 'NONE',  ( -0.000000000000000000, 1.000000000000000000, -0.000000000000000000 ) ) ;
#24910=CARTESIAN_POINT ( 'NONE',  ( 99.14382582708707048, 123.1000000010924822, 2.066987299999979211 ) ) ;
#24949=CARTESIAN_POINT ( 'NONE',  ( 101.0355339059327378, 123.9500000000000028, -2.499999999999997780 ) ) ;
#24962=ORIENTED_EDGE ( 'NONE', *, *, #19448, .T. ) ;
#24996=CARTESIAN_POINT ( 'NONE',  ( 100.8561741729129295, 124.0000000010925021, 2.066987299999979211 ) ) ;
#25010=( BOUNDED_CURVE ( )  B_SPLINE_CURVE ( 2, ( #9053, #2920, #24440, #4781, #9190, #26881, #3068, #22168, #2646 ),
 .UNSPECIFIED., .F., .T. ) 
 B_SPLINE_CURVE_WITH_KNOTS ( ( 3, 2, 2, 2, 3 ),
 ( 0.08333333333333307891, 0.1249999999999999167, 0.1666666666666667407, 0.2083333333333335924, 0.2500000000000004441 ),
 .UNSPECIFIED. ) 
 CURVE ( )  GEOMETRIC_REPRESENTATION_ITEM ( )  RATIONAL_B_SPLINE_CURVE ( ( 1.000000000000000444, 0.9238795325112862944, 1.000000000000000000, 0.9238795325112867385, 1.000000000000000000, 0.9238795325112867385, 1.000000000000000000, 0.9238795325112859613, 1.000000000000000888 ) ) 
 REPRESENTATION_ITEM ( '' )  );
#25016=DIRECTION ( 'NONE',  ( 0.000000000000000000, 0.000000000000000000, 1.000000000000000000 ) ) ;
#25051=CARTESIAN_POINT ( 'NONE',  ( 102.0669872999999939, 123.4000000010924936, -0.8561741729129507261 ) ) ;
#25092=CARTESIAN_POINT ( 'NONE',  ( 98.23223304703363112, 124.1000000000000085, -1.767766952966370209 ) ) ;
#25130=CARTESIAN_POINT ( 'NONE',  ( 99.14382582708707048, 124.4000000010924794, -2.066987299999999195 ) ) ;
#25163=CIRCLE ( 'NONE', #21082, 10.50000000000001599 ) ;
#25177=CARTESIAN_POINT ( 'NONE',  ( 98.96446609406727646, 123.6500000021849530, 2.499999999999977796 ) ) ;
#25185=CARTESIAN_POINT ( 'NONE',  ( 102.0669872999999797, 122.5500000010924850, -9.794112055954760458E-15 ) ) ;
#25204=CARTESIAN_POINT ( 'NONE',  ( 102.4999999999999858, 122.9999999999999858, 0.3272492347489319164 ) ) ;
#25227=CARTESIAN_POINT ( 'NONE',  ( 97.50000000000000000, 123.4500000000000028, 1.035533905932725096 ) ) ;
#25235=CARTESIAN_POINT ( 'NONE',  ( 99.99999999999998579, 128.0000000000000000, -0.5000000000000138778 ) ) ;
#25277=DIRECTION ( 'NONE',  ( 0.000000000000000000, 0.000000000000000000, -1.000000000000000000 ) ) ;
#25295=FACE_BOUND ( 'NONE', #26299, .T. ) ;
#25315=CARTESIAN_POINT ( 'NONE',  ( 102.4999999999999716, 123.9500000021849502, -1.035533905932742638 ) ) ;
#25323=CARTESIAN_POINT ( 'NONE',  ( 99.14382582708707048, 123.0000000010925021, -2.066987299999999195 ) ) ;
#25370=CARTESIAN_POINT ( 'NONE',  ( 99.14382582708707048, 124.1000000010924964, 2.066987299999979211 ) ) ;
#25373=PRODUCT_CONTEXT ( 'NONE', #10768, 'mechanical' ) ;
#25382=LINE ( 'NONE', #17084, #17994 ) ;
#25421=EDGE_LOOP ( 'NONE', ( #26878, #2343 ) ) ;
#25441=CARTESIAN_POINT ( 'NONE',  ( 99.99999999999998579, 123.6000000000000085, 2.499999999999978684 ) ) ;
#25538=ORIENTED_EDGE ( 'NONE', *, *, #324, .T. ) ;
#25556=CARTESIAN_POINT ( 'NONE',  ( 101.9373566580610628, 122.9999999999999858, -1.366919386427927874 ) ) ;
#25597=CARTESIAN_POINT ( 'NONE',  ( 99.14382582708707048, 124.1000000010924964, 2.066987299999979211 ) ) ;
#25601=ORIENTED_EDGE ( 'NONE', *, *, #27805, .F. ) ;
#25655=CYLINDRICAL_SURFACE ( 'NONE', #10193, 0.5000000000000086597 ) ;
#25689=VERTEX_POINT ( 'NONE', #18579 ) ;
#25736=CARTESIAN_POINT ( 'NONE',  ( 99.14382582708707048, 122.8000000010924708, -2.066987299999999195 ) ) ;
#25742=VECTOR ( 'NONE', #1035, 1000.000000000000000 ) ;
#25843=EDGE_CURVE ( 'NONE', #3824, #3142, #25163, .T. ) ;
#25853=DIRECTION ( 'NONE',  ( 0.000000000000000000, 0.000000000000000000, -1.000000000000000000 ) ) ;
#25879=CARTESIAN_POINT ( 'NONE',  ( 99.99999999999998579, 138.0000000000000000, -11.50000000000002309 ) ) ;
#25892=EDGE_CURVE ( 'NONE', #4566, #26480, #19621, .T. ) ;
#25931=CARTESIAN_POINT ( 'NONE',  ( 97.94614682514237813, 122.9999999999999858, -0.2688731231943997102 ) ) ;
#25969=CARTESIAN_POINT ( 'NONE',  ( 99.99999999999998579, 123.7500000010924737, -2.066987299999998751 ) ) ;
#26053=EDGE_CURVE ( 'NONE', #26480, #20976, #3342, .T. ) ;
#26159=CARTESIAN_POINT ( 'NONE',  ( 99.99999999999998579, 124.3999999999999915, 2.499999999999978684 ) ) ;
#26223=EDGE_CURVE ( 'NONE', #1875, #15313, #1009, .T. ) ;
#26299=EDGE_LOOP ( 'NONE', ( #10988, #24663 ) ) ;
#26346=CARTESIAN_POINT ( 'NONE',  ( 99.99999999999998579, 130.0000000000000000, -5.204170427930421283E-15 ) ) ;
#26389=CARTESIAN_POINT ( 'NONE',  ( 102.0669872999999939, 124.4000000010924651, -0.8561741729129507261 ) ) ;
#26400=ORIENTED_EDGE ( 'NONE', *, *, #3840, .T. ) ;
#26447=VECTOR ( 'NONE', #9092, 999.9999999999998863 ) ;
#26452=CARTESIAN_POINT ( 'NONE',  ( 98.96446609406726225, 124.0499999999999829, -2.499999999999998668 ) ) ;
#26480=VERTEX_POINT ( 'NONE', #9012 ) ;
#26530=CARTESIAN_POINT ( 'NONE',  ( 101.4615807364564546, 124.2500000010924737, 1.461580736456455476 ) ) ;
#26542=CARTESIAN_POINT ( 'NONE',  ( 102.0669873000000081, 123.5000000010924737, 0.8561741729129311862 ) ) ;
#26565=ORIENTED_EDGE ( 'NONE', *, *, #15657, .F. ) ;
#26588=CARTESIAN_POINT ( 'NONE',  ( 97.93301270000000613, 124.5000000010924879, -0.8561741729129506151 ) ) ;
#26607=DIRECTION ( 'NONE',  ( -0.000000000000000000, -1.000000000000000000, -0.000000000000000000 ) ) ;
#26645=EDGE_CURVE ( 'NONE', #3142, #3824, #23821, .T. ) ;
#26683=VECTOR ( 'NONE', #22474, 1000.000000000000000 ) ;
#26726=ORIENTED_EDGE ( 'NONE', *, *, #5269, .F. ) ;
#26731=CARTESIAN_POINT ( 'NONE',  ( 99.99999999999998579, 124.3500000010924822, -2.066987299999998751 ) ) ;
#26741=ORIENTED_EDGE ( 'NONE', *, *, #17674, .F. ) ;
#26767=ORIENTED_EDGE ( 'NONE', *, *, #24509, .F. ) ;
#26778=CARTESIAN_POINT ( 'NONE',  ( 102.0669872999999797, 124.1500000010924794, -9.794112055954760458E-15 ) ) ;
#26817=CARTESIAN_POINT ( 'NONE',  ( 99.99999999999998579, 138.0000000000000000, -10.50000000000002132 ) ) ;
#26844=AXIS2_PLACEMENT_3D ( 'NONE', #8635, #24028, #23608 ) ;
#26866=CARTESIAN_POINT ( 'NONE',  ( 101.7677669529663547, 122.4000000021849530, -1.767766952966370209 ) ) ;
#26878=ORIENTED_EDGE ( 'NONE', *, *, #9818, .T. ) ;
#26879=CARTESIAN_POINT ( 'NONE',  ( 102.0669872999999797, 123.3500000010924680, -9.794112055954760458E-15 ) ) ;
#26881=CARTESIAN_POINT ( 'NONE',  ( 102.4999999999999858, 123.8500000021849416, 1.035533905932722876 ) ) ;
#26910=ORIENTED_EDGE ( 'NONE', *, *, #8481, .F. ) ;
#26925=CARTESIAN_POINT ( 'NONE',  ( 102.4999999999999858, 123.1500000021849672, -1.035533905932742638 ) ) ;
#26927=CARTESIAN_POINT ( 'NONE',  ( 99.99999999999998579, 128.0000000000000000, -2.500000000000013767 ) ) ;
#26961=DIRECTION ( 'NONE',  ( 0.000000000000000000, 0.000000000000000000, 1.000000000000000000 ) ) ;
#26989=CARTESIAN_POINT ( 'NONE',  ( 98.96446609406724804, 123.2499999999999716, -2.499999999999993339 ) ) ;
#27004=ORIENTED_EDGE ( 'NONE', *, *, #3075, .F. ) ;
#27006=CARTESIAN_POINT ( 'NONE',  ( 102.0669872999999939, 122.6000000010924964, -0.8561741729129507261 ) ) ;
#27101=CARTESIAN_POINT ( 'NONE',  ( 98.96446609406724804, 123.3500000021849274, -2.499999999999996447 ) ) ;
#27105=CARTESIAN_POINT ( 'NONE',  ( 97.50000000000000000, 124.9500000000000028, -1.035533905932742416 ) ) ;
#27152=CARTESIAN_POINT ( 'NONE',  ( 101.4615807364564546, 123.4500000010924765, -1.461580736456474794 ) ) ;
#27206=DIRECTION ( 'NONE',  ( 0.000000000000000000, -1.000000000000000000, 0.000000000000000000 ) ) ;
#27245=CARTESIAN_POINT ( 'NONE',  ( 101.4615807364564546, 122.8500000010924680, -1.461580736456474794 ) ) ;
#27256=AXIS2_PLACEMENT_3D ( 'NONE', #9065, #9204, #14279 ) ;
#27261=ADVANCED_FACE ( 'NONE', ( #1439 ), #10097, .T. ) ;
#27266=EDGE_LOOP ( 'NONE', ( #11139, #8268, #16984, #22322 ) ) ;
#27272=VECTOR ( 'NONE', #22490, 999.9999999999998863 ) ;
#27286=CARTESIAN_POINT ( 'NONE',  ( 98.23223304703363112, 122.6000000021849559, -1.767766952966370209 ) ) ;
#27300=ORIENTED_EDGE ( 'NONE', *, *, #4279, .F. ) ;
#27342=CARTESIAN_POINT ( 'NONE',  ( 98.53841926354351699, 124.0500000010924708, 1.461580736456455920 ) ) ;
#27382=CARTESIAN_POINT ( 'NONE',  ( 101.7677669529663547, 123.7000000000000028, 1.767766952966350891 ) ) ;
#27418=CARTESIAN_POINT ( 'NONE',  ( 97.93301269999999192, 123.8000000010924850, 0.8561741729129329626 ) ) ;
#27426=CARTESIAN_POINT ( 'NONE',  ( 99.99999999999998579, 138.0000000000000000, -5.204170427930421283E-15 ) ) ;
#27466=CARTESIAN_POINT ( 'NONE',  ( 99.99999999999998579, 137.0000000000000000, 12.50000000000001066 ) ) ;
#27469=CARTESIAN_POINT ( 'NONE',  ( 99.99999999999998579, 124.1000000021849416, -2.499999999999997780 ) ) ;
#27477=CARTESIAN_POINT ( 'NONE',  ( 99.14382582708707048, 123.8000000010924850, -2.066987299999999195 ) ) ;
#27518=CARTESIAN_POINT ( 'NONE',  ( 102.0669872999999939, 123.5000000010924595, 0.8561741729129311862 ) ) ;
#27520=EDGE_CURVE ( 'NONE', #18580, #1596, #4967, .T. ) ;
#27562=CARTESIAN_POINT ( 'NONE',  ( 102.4842213106612547, 122.9999999999999716, -0.1886707679707059215 ) ) ;
#27575=B_SPLINE_CURVE_WITH_KNOTS ( 'NONE', 3,
 ( #2283, #11366, #10941, #20088, #566, #22085, #4414, #19653, #9248, #25931, #135, #8821, #16075, #9530 ),
 .UNSPECIFIED., .F., .F.,
 ( 4, 2, 2, 2, 2, 2, 4 ),
 ( 1.718536712070695008E-16, 0.0008152643689839393290, 0.001222896553475838087, 0.001630528737967736628, 0.002038160922459635385, 0.002445793106951534360, 0.003261057475935332309 ),
 .UNSPECIFIED. ) ;
#27582=FILL_AREA_STYLE_COLOUR ( '', #23193 ) ;
#27604=CARTESIAN_POINT ( 'NONE',  ( 98.96446609406727646, 124.1500000021849672, -2.499999999999997780 ) ) ;
#27614=CARTESIAN_POINT ( 'NONE',  ( 97.93301270000000613, 123.1500000010924651, -9.540979117872439019E-15 ) ) ;
#27647=AXIS2_PLACEMENT_3D ( 'NONE', #18747, #16603, #6060 ) ;
#27650=CARTESIAN_POINT ( 'NONE',  ( 99.99999999999998579, 123.7000000021849502, 2.499999999999978684 ) ) ;
#27668=CARTESIAN_POINT ( 'NONE',  ( 97.50000000000000000, 124.2500000021849900, -1.035533905932742416 ) ) ;
#27702=CARTESIAN_POINT ( 'NONE',  ( 101.6707202882716388, 122.9999999999999574, -1.633471722151653704 ) ) ;
#27704=EDGE_LOOP ( 'NONE', ( #22915, #9006 ) ) ;
#27723=DIRECTION ( 'NONE',  ( -0.000000000000000000, -1.000000000000000000, -0.000000000000000000 ) ) ;
#27744=DIRECTION ( 'NONE',  ( 0.000000000000000000, 0.000000000000000000, -1.000000000000000000 ) ) ;
#27750=CARTESIAN_POINT ( 'NONE',  ( 102.0669872999999797, 123.5500000010924708, -9.794112055954760458E-15 ) ) ;
#27753=DIRECTION ( 'NONE',  ( 0.000000000000000000, 0.000000000000000000, -1.000000000000000000 ) ) ;
#27805=EDGE_CURVE ( 'NONE', #24651, #487, #11351, .T. ) ;
#27826=CONICAL_SURFACE ( 'NONE', #6870, 12.50000000000001599, 0.7853981633974491672 ) ;
#27839=EDGE_LOOP ( 'NONE', ( #23525, #17527, #5482, #5375 ) ) ;
#27886=CARTESIAN_POINT ( 'NONE',  ( 97.93301269999999192, 123.2000000010924765, 0.8561741729129329626 ) ) ;
#27927=CARTESIAN_POINT ( 'NONE',  ( 101.7677669529663547, 123.0999999999999943, -1.767766952966370209 ) ) ;
#27944=CARTESIAN_POINT ( 'NONE',  ( 99.99999999999998579, 128.0000000000000000, -5.204170427930421283E-15 ) ) ;
#28021=DIRECTION ( 'NONE',  ( 0.000000000000000000, -0.7071067811865482389, -0.7071067811865469066 ) ) ;
#28022=AXIS2_PLACEMENT_3D ( 'NONE', #1784, #27723, #25853 ) ;
#28109=CARTESIAN_POINT ( 'NONE',  ( 99.99999999999998579, 130.0000000000000000, 10.50000000000001066 ) ) ;
#28114=CARTESIAN_POINT ( 'NONE',  ( 102.0669872999999797, 123.5500000010924708, -9.794112055954760458E-15 ) ) ;
#28138=CARTESIAN_POINT ( 'NONE',  ( 99.99999999999998579, 124.7999999999999972, -2.499999999999997780 ) ) ;
#28189=CYLINDRICAL_SURFACE ( 'NONE', #13862, 2.500000000000008882 ) ;
#28200=DIRECTION ( 'NONE',  ( 0.000000000000000000, 0.000000000000000000, 1.000000000000000000 ) ) ;
ENDSEC;
END-ISO-10303-21;
